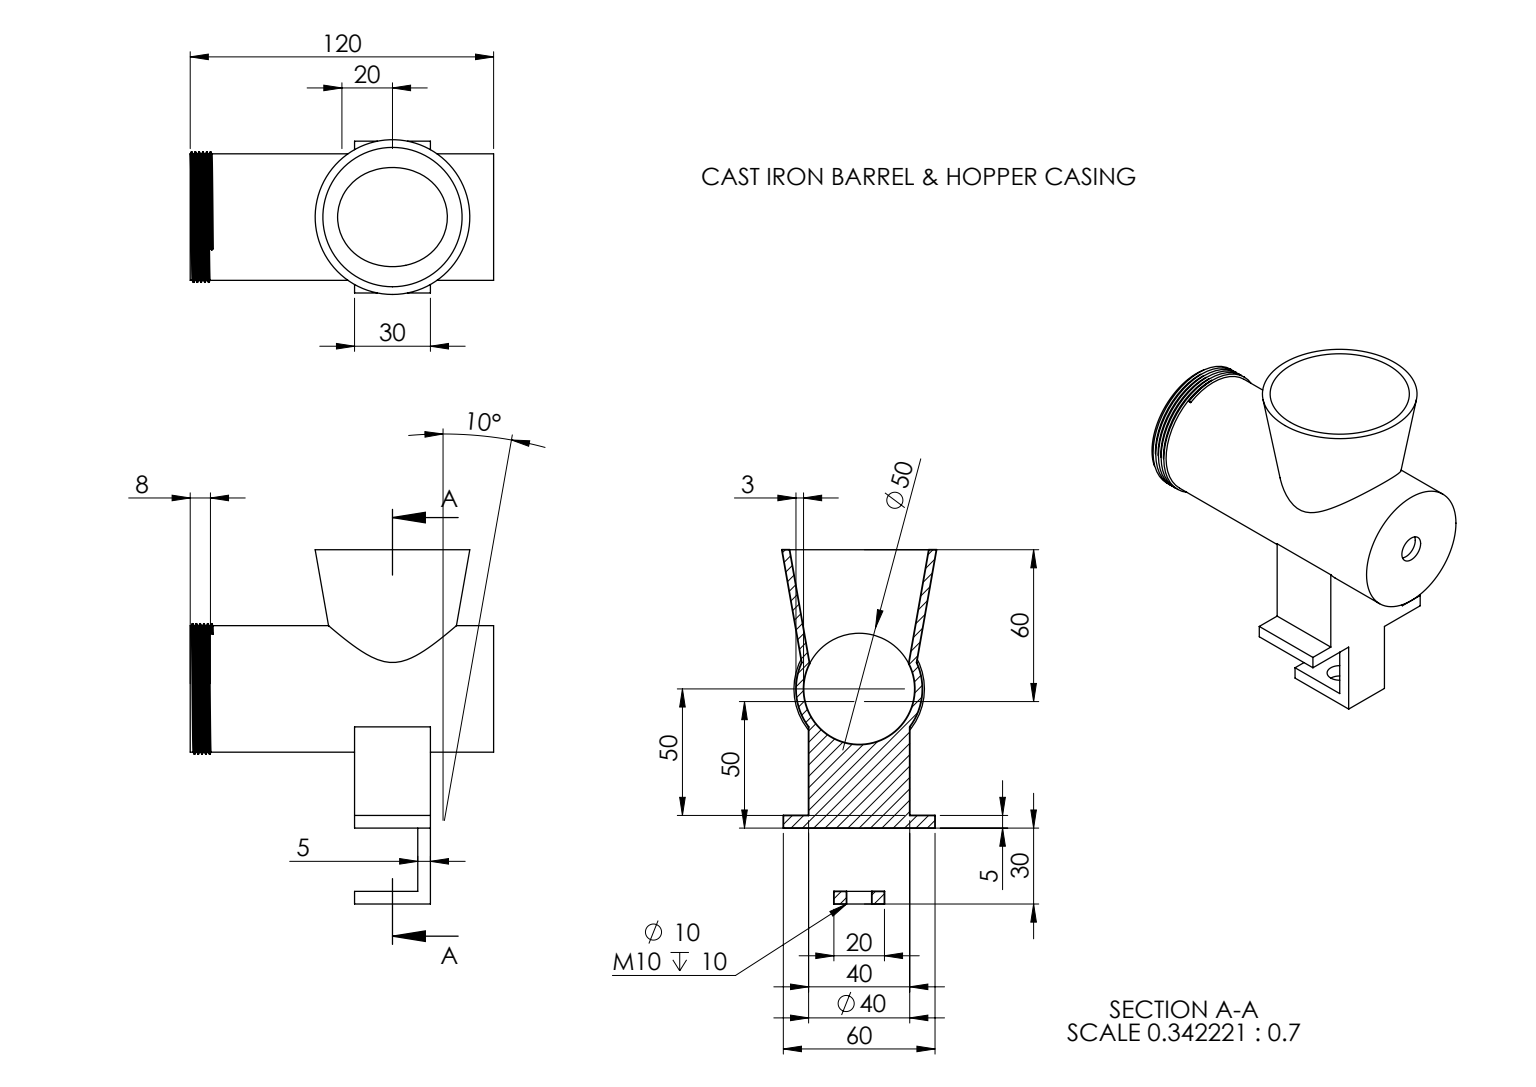
ISO-10303-21;
HEADER;
FILE_DESCRIPTION (('STEP AP214'),
    '1' );
FILE_NAME ('Cast Iron Barrel & Hopper Casing.step',
    '2026-10-22T10:02:39',
    ( '' ),
    ( '' ),
    'SwSTEP 2.0',
    'SolidWorks 2026',
    '' );
FILE_SCHEMA (( 'AUTOMOTIVE_DESIGN' ));
ENDSEC;

DATA;
#1=CARTESIAN_POINT ( 'NONE',  ( -15.00000000000000000, 55.00000000000000000, -20.00000000000000000 ) ) ;
#5=CARTESIAN_POINT ( 'NONE',  ( -21.63041020058595976, 76.92929161012460781, 1.799941901431467484 ) ) ;
#6=VECTOR ( 'NONE', #483, 1000.000000000000000 ) ;
#10=CARTESIAN_POINT ( 'NONE',  ( -15.00000000000000000, 5.000000000000000000, 20.00000000000000000 ) ) ;
#11=VERTEX_POINT ( 'NONE', #2092 ) ;
#13=CARTESIAN_POINT ( 'NONE',  ( -73.34375000204839523, 73.25176868561975141, -18.25176868561974430 ) ) ;
#30=VERTEX_POINT ( 'NONE', #8511 ) ;
#31=CARTESIAN_POINT ( 'NONE',  ( -76.62500000409677625, 55.00000000000000000, 24.99999999999999645 ) ) ;
#39=LINE ( 'NONE', #6477, #6145 ) ;
#41=CARTESIAN_POINT ( 'NONE',  ( -74.00000000204839523, 29.18810118750000981, 10.69163855873950020 ) ) ;
#44=CARTESIAN_POINT ( 'NONE',  ( -76.71875000204839523, 29.18810118750000271, 4.741568889096522788E-15 ) ) ;
#49=DIRECTION ( 'NONE',  ( 1.000000000000000000, 0.000000000000000000, 0.000000000000000000 ) ) ;
#50=LINE ( 'NONE', #11190, #9309 ) ;
#51=CARTESIAN_POINT ( 'NONE',  ( -78.03125000000002842, 79.99999999999992895, 10.35533905932734378 ) ) ;
#53=CARTESIAN_POINT ( 'NONE',  ( -79.25000000000000000, 55.00000000000000000, 24.99999999999999645 ) ) ;
#62=CARTESIAN_POINT ( 'NONE',  ( -19.12261397941723473, 74.85860496676178855, 9.489298872914485372 ) ) ;
#64=EDGE_CURVE ( 'NONE', #4200, #8679, #1605, .T. ) ;
#71=CARTESIAN_POINT ( 'NONE',  ( -71.59560441781462714, 80.81189881250000440, 6.916273779317701376 ) ) ;
#73=ADVANCED_FACE ( 'NONE', ( #817 ), #4433, .F. ) ;
#93=CARTESIAN_POINT ( 'NONE',  ( 9.999999999999994671, -24.99999999999999645, 10.00000000000000000 ) ) ;
#98=CARTESIAN_POINT ( 'NONE',  ( -71.75000000204838102, 80.81189881250000440, -10.69163855873948954 ) ) ;
#99=CARTESIAN_POINT ( 'NONE',  ( 3.371861548457865722E-15, 110.0000000000000000, -27.53333900685068869 ) ) ;
#101=CARTESIAN_POINT ( 'NONE',  ( 0.000000000000000000, -24.99999999999999645, -5.000000000000000000 ) ) ;
#104=ORIENTED_EDGE ( 'NONE', *, *, #11406, .F. ) ;
#105=CARTESIAN_POINT ( 'NONE',  ( -77.65625000204839523, 73.25176868561975141, -18.25176868561974430 ) ) ;
#107=CARTESIAN_POINT ( 'NONE',  ( 24.10175047695886619, 78.98596163070220655, -7.059706225875322261 ) ) ;
#109=VECTOR ( 'NONE', #311, 1000.000000000000000 ) ;
#111=EDGE_CURVE ( 'NONE', #9073, #8979, #3345, .T. ) ;
#112=DIRECTION ( 'NONE',  ( 0.000000000000000000, -0.000000000000000000, 1.000000000000000000 ) ) ;
#115=VECTOR ( 'NONE', #7085, 1000.000000000000000 ) ;
#116=CARTESIAN_POINT ( 'NONE',  ( -78.31250000000000000, 72.67766952966368876, -17.67766952966368876 ) ) ;
#120=DIRECTION ( 'NONE',  ( 1.000000000000000000, 0.000000000000000000, -0.000000000000000000 ) ) ;
#122=SHAPE_DEFINITION_REPRESENTATION ( #1837, #423 ) ;
#124=CARTESIAN_POINT ( 'NONE',  ( -10.64432325360710152, 68.67941443230903076, -17.23560473394323367 ) ) ;
#133=PRODUCT_DEFINITION ( 'UNKNOWN', '', #852, #2465 ) ;
#134=CARTESIAN_POINT ( 'NONE',  ( -76.71875000204839523, 29.18810118750000271, 4.741568889096522788E-15 ) ) ;
#135=CARTESIAN_POINT ( 'NONE',  ( -15.00000000000000355, 5.000000000000000000, -29.99999999999999289 ) ) ;
#138=ORIENTED_EDGE ( 'NONE', *, *, #9495, .F. ) ;
#140=EDGE_CURVE ( 'NONE', #7402, #8679, #2318, .T. ) ;
#147=CARTESIAN_POINT ( 'NONE',  ( -73.34375000409679046, 30.00000000000001421, 10.35533905932739174 ) ) ;
#148=DIRECTION ( 'NONE',  ( -1.000000000000000000, -0.000000000000000000, -0.000000000000000000 ) ) ;
#153=DIRECTION ( 'NONE',  ( 0.000000000000000000, -0.000000000000000000, 1.000000000000000000 ) ) ;
#160=ORIENTED_EDGE ( 'NONE', *, *, #1242, .F. ) ;
#164=FACE_BOUND ( 'NONE', #3650, .T. ) ;
#165=CARTESIAN_POINT ( 'NONE',  ( -12.37866201454132487, 69.98577131611273217, -20.01755997183146718 ) ) ;
#168=CARTESIAN_POINT ( 'NONE',  ( -78.59375000204839523, 55.00000000000000000, 25.81189881249999729 ) ) ;
#171=CARTESIAN_POINT ( 'NONE',  ( 3.392634454741613848, 65.79950035100726780, -22.54765914078175015 ) ) ;
#178=CARTESIAN_POINT ( 'NONE',  ( -15.00000000000000355, 0.000000000000000000, -29.99999999999999289 ) ) ;
#179=VECTOR ( 'NONE', #1295, 1000.000000000000000 ) ;
#182=FACE_OUTER_BOUND ( 'NONE', #3755, .T. ) ;
#187=CARTESIAN_POINT ( 'NONE',  ( -7.638500494831339971, 67.00046308197731548, 18.44294210305378456 ) ) ;
#191=FACE_OUTER_BOUND ( 'NONE', #2836, .T. ) ;
#193=VERTEX_POINT ( 'NONE', #2983 ) ;
#196=CARTESIAN_POINT ( 'NONE',  ( -78.68750000204839523, 65.69163855873949842, 25.81189881250000440 ) ) ;
#204=ORIENTED_EDGE ( 'NONE', *, *, #9495, .T. ) ;
#205=CARTESIAN_POINT ( 'NONE',  ( -71.93750000204838102, 44.30836144126049447, -25.81189881249999019 ) ) ;
#208=FACE_OUTER_BOUND ( 'NONE', #5773, .T. ) ;
#214=CARTESIAN_POINT ( 'NONE',  ( -75.87500000409677625, 55.00000000000000000, -24.99999999999999645 ) ) ;
#218=ORIENTED_EDGE ( 'NONE', *, *, #5065, .F. ) ;
#230=CARTESIAN_POINT ( 'NONE',  ( -71.84375000204838102, 73.25176868561975141, -18.25176868561974430 ) ) ;
#233=CARTESIAN_POINT ( 'NONE',  ( -76.06250000409679046, 37.32233047033631124, -17.67766952966368166 ) ) ;
#234=ORIENTED_EDGE ( 'NONE', *, *, #5652, .T. ) ;
#235=CARTESIAN_POINT ( 'NONE',  ( 23.67201755683229081, 78.62200754200915753, -8.225812365109568702 ) ) ;
#249=EDGE_LOOP ( 'NONE', ( #1338, #6982, #2879, #8696 ) ) ;
#254=CARTESIAN_POINT ( 'NONE',  ( -75.87500000204839523, 80.81189881250001861, 10.69163855873948599 ) ) ;
#259=ORIENTED_EDGE ( 'NONE', *, *, #6814, .T. ) ;
#261=CARTESIAN_POINT ( 'NONE',  ( -73.71875000204839523, 29.18810118750000271, 4.741568889096522788E-15 ) ) ;
#270=CARTESIAN_POINT ( 'NONE',  ( -76.34375000409679046, 30.00000000000001421, 10.35533905932739174 ) ) ;
#272=CARTESIAN_POINT ( 'NONE',  ( -72.06435441788595142, 79.99999999999991473, 6.698726029249561620 ) ) ;
#278=PLANE ( 'NONE',  #4388 ) ;
#279=CARTESIAN_POINT ( 'NONE',  ( -15.00000000000000000, -24.99999999999999645, 10.00000000000000000 ) ) ;
#292=CARTESIAN_POINT ( 'NONE',  ( -73.62500000204842365, 29.18810118750000626, -10.69163855873949309 ) ) ;
#294=DIRECTION ( 'NONE',  ( -1.000000000000000000, 0.000000000000000000, -0.000000000000000000 ) ) ;
#296=CARTESIAN_POINT ( 'NONE',  ( 0.000000000000000000, 0.000000000000000000, 10.00000000000000000 ) ) ;
#303=CARTESIAN_POINT ( 'NONE',  ( -77.28124999999998579, 30.00000000000000355, -10.35533905932738108 ) ) ;
#305=CARTESIAN_POINT ( 'NONE',  ( -77.00000000000000000, 55.00000000000000000, -24.99999999999999645 ) ) ;
#309=CARTESIAN_POINT ( 'NONE',  ( -2.905210441188253778, 65.30173033721455056, 19.43922460838591348 ) ) ;
#311=DIRECTION ( 'NONE',  ( 1.000000000000000000, 0.000000000000000000, 0.000000000000000000 ) ) ;
#312=ORIENTED_EDGE ( 'NONE', *, *, #8953, .F. ) ;
#313=DIRECTION ( 'NONE',  ( 0.000000000000000000, 0.000000000000000000, -1.000000000000000000 ) ) ;
#317=CARTESIAN_POINT ( 'NONE',  ( -73.90625000204839523, 36.74823131438026280, 18.25176868561974786 ) ) ;
#333=CARTESIAN_POINT ( 'NONE',  ( -72.31250000000007105, 72.67766952966360350, -17.67766952966359995 ) ) ;
#343=DIRECTION ( 'NONE',  ( 0.000000000000000000, 1.000000000000000000, 0.000000000000000000 ) ) ;
#346=CARTESIAN_POINT ( 'NONE',  ( -3.398726575883826762, 65.81855960629934543, 22.53824819929336698 ) ) ;
#350=CARTESIAN_POINT ( 'NONE',  ( -78.21875000409679046, 65.35533905932737753, 24.99999999999999645 ) ) ;
#352=CARTESIAN_POINT ( 'NONE',  ( 12.39308895597016047, 69.98013642987091032, -20.04675360703169318 ) ) ;
#355=AXIS2_PLACEMENT_3D ( 'NONE', #11527, #8791, #3333 ) ;
#360=CARTESIAN_POINT ( 'NONE',  ( -74.56250000000000000, 37.32233047033631124, 17.67766952966369232 ) ) ;
#367=DIRECTION ( 'NONE',  ( -0.000000000000000000, -1.000000000000000000, -0.000000000000000000 ) ) ;
#372=CARTESIAN_POINT ( 'NONE',  ( 39.99999999999999289, 55.00000000000000000, 0.000000000000000000 ) ) ;
#373=CARTESIAN_POINT ( 'NONE',  ( -75.96875000204839523, 73.25176868561975141, 18.25176868561974075 ) ) ;
#377=CARTESIAN_POINT ( 'NONE',  ( -75.03125000204839523, 36.74823131438024859, -18.25176868561973720 ) ) ;
#381=CARTESIAN_POINT ( 'NONE',  ( -15.00000000000000355, 0.000000000000000000, 30.00000000000000711 ) ) ;
#384=CARTESIAN_POINT ( 'NONE',  ( -74.00000000204839523, 44.30836144126052289, 25.81189881250000795 ) ) ;
#385=CARTESIAN_POINT ( 'NONE',  ( -80.00000000000000000, 55.00000000000000000, 24.99999999999999645 ) ) ;
#388=VERTEX_POINT ( 'NONE', #6780 ) ;
#399=CIRCLE ( 'NONE', #11681, 24.99999999999999645 ) ;
#408=CARTESIAN_POINT ( 'NONE',  ( -75.31250000204839523, 29.18810118750000981, 10.69163855873950020 ) ) ;
#412=CARTESIAN_POINT ( 'NONE',  ( -77.65625000409677625, 30.00000000000000355, -10.35533905932738108 ) ) ;
#419=CARTESIAN_POINT ( 'NONE',  ( -73.71875000000005684, 79.99999999999987210, -10.35533905932732424 ) ) ;
#421=CARTESIAN_POINT ( 'NONE',  ( -77.09374999999998579, 44.64466094067260826, -24.99999999999998934 ) ) ;
#423=SHAPE_REPRESENTATION ( 'Cast Iron Barrel & Hopper Casing', ( #4738 ), #3015 ) ;
#426=EDGE_CURVE ( 'NONE', #7502, #11, #9516, .T. ) ;
#427=ADVANCED_FACE ( 'NONE', ( #5819, #10408 ), #5935, .F. ) ;
#431=CARTESIAN_POINT ( 'NONE',  ( 10.64984185237921466, 68.68279778901450072, -17.23294504368761793 ) ) ;
#433=CARTESIAN_POINT ( 'NONE',  ( -78.87500000204839523, 65.69163855873949842, 25.81189881250000084 ) ) ;
#436=CARTESIAN_POINT ( 'NONE',  ( -72.68750000204839523, 65.69163855873949842, 25.81189881250000440 ) ) ;
#437=ADVANCED_FACE ( 'NONE', ( #8976 ), #2509, .T. ) ;
#454=CARTESIAN_POINT ( 'NONE',  ( -73.62500000409677625, 55.00000000000000000, 24.99999999999999645 ) ) ;
#464=FACE_OUTER_BOUND ( 'NONE', #2972, .T. ) ;
#465=DIRECTION ( 'NONE',  ( 0.000000000000000000, 0.000000000000000000, 1.000000000000000000 ) ) ;
#466=CARTESIAN_POINT ( 'NONE',  ( -77.09375000204839523, 55.00000000000000000, 25.81189881249999729 ) ) ;
#467=CARTESIAN_POINT ( 'NONE',  ( -11.05058114698192107, 69.12285606448547526, 20.64999657351882689 ) ) ;
#470=CARTESIAN_POINT ( 'NONE',  ( -76.34375000409680467, 30.00000000000001421, 10.35533905932739174 ) ) ;
#474=CARTESIAN_POINT ( 'NONE',  ( -75.21875000000007105, 79.99999999999990052, -10.35533905932733134 ) ) ;
#481=CARTESIAN_POINT ( 'NONE',  ( -72.21875000000001421, 80.00000000000001421, -10.35533905932737753 ) ) ;
#483=DIRECTION ( 'NONE',  ( -0.000000000000000000, -0.000000000000000000, -1.000000000000000000 ) ) ;
#485=EDGE_CURVE ( 'NONE', #7813, #9573, #2446, .T. ) ;
#488=LINE ( 'NONE', #11560, #10630 ) ;
#492=CARTESIAN_POINT ( 'NONE',  ( 21.70367235178696319, 76.99085433373973331, 0.7325029477543631984 ) ) ;
#493=CARTESIAN_POINT ( 'NONE',  ( -77.84375000204839523, 73.25176868561975141, -18.25176868561974430 ) ) ;
#494=VERTEX_POINT ( 'NONE', #7845 ) ;
#495=CARTESIAN_POINT ( 'NONE',  ( -72.03125000204839523, 36.74823131438024859, -18.25176868561973720 ) ) ;
#500=ORIENTED_EDGE ( 'NONE', *, *, #3520, .F. ) ;
#502=ORIENTED_EDGE ( 'NONE', *, *, #10815, .T. ) ;
#523=CARTESIAN_POINT ( 'NONE',  ( -79.06250000204840944, 80.81189881250000440, -10.69163855873948954 ) ) ;
#524=CARTESIAN_POINT ( 'NONE',  ( -1.708601562010274133, 65.50638515368892456, 22.68572929305231867 ) ) ;
#526=ORIENTED_EDGE ( 'NONE', *, *, #1693, .F. ) ;
#527=CARTESIAN_POINT ( 'NONE',  ( -74.37500000409677625, 55.00000000000000000, -24.99999999999999645 ) ) ;
#530=AXIS2_PLACEMENT_3D ( 'NONE', #8639, #9703, #5223 ) ;
#538=CARTESIAN_POINT ( 'NONE',  ( -74.75000000000000000, 55.00000000000000000, 24.99999999999999645 ) ) ;
#542=EDGE_CURVE ( 'NONE', #5255, #5411, #11153, .T. ) ;
#546=VERTEX_POINT ( 'NONE', #9861 ) ;
#547=CARTESIAN_POINT ( 'NONE',  ( 2.917962331683024768, 65.29045701389995315, -19.44540138122387773 ) ) ;
#549=ORIENTED_EDGE ( 'NONE', *, *, #6671, .F. ) ;
#552=CARTESIAN_POINT ( 'NONE',  ( -75.40625000409677625, 80.00000000000001421, 10.35533905932737397 ) ) ;
#565=CARTESIAN_POINT ( 'NONE',  ( -74.18750000204838102, 44.30836144126053000, 25.81189881250000795 ) ) ;
#580=CARTESIAN_POINT ( 'NONE',  ( -77.46875000204839523, 80.81189881250000440, -1.580522963032174394E-15 ) ) ;
#584=CARTESIAN_POINT ( 'NONE',  ( -75.12500000409677625, 55.00000000000000000, 24.99999999999999645 ) ) ;
#585=DIRECTION ( 'NONE',  ( -1.000000000000000000, -0.000000000000000000, -0.000000000000000000 ) ) ;
#586=CARTESIAN_POINT ( 'NONE',  ( -71.56250000409677625, 37.32233047033631124, -17.67766952966368166 ) ) ;
#592=AXIS2_PLACEMENT_3D ( 'NONE', #1916, #1680, #10056 ) ;
#594=CARTESIAN_POINT ( 'NONE',  ( 39.99999999999999289, 55.00000000000000000, 0.000000000000000000 ) ) ;
#598=CARTESIAN_POINT ( 'NONE',  ( -78.03125000204838102, 55.00000000000000000, -25.81189881249999729 ) ) ;
#610=VECTOR ( 'NONE', #11628, 1000.000000000000000 ) ;
#611=CARTESIAN_POINT ( 'NONE',  ( 12.31292331232940640, 69.75642766769821890, 16.32415115763334867 ) ) ;
#612=CARTESIAN_POINT ( 'NONE',  ( -72.12500000204839523, 44.30836144126049447, -25.81189881249999019 ) ) ;
#625=CARTESIAN_POINT ( 'NONE',  ( -77.75000000204839523, 80.81189881250001861, -10.69163855873949132 ) ) ;
#630=( BOUNDED_CURVE ( )  B_SPLINE_CURVE ( 2, ( #7577, #9479, #6681, #10311, #8593, #2108, #3973, #5782, #1209 ),
 .UNSPECIFIED., .F., .T. ) 
 B_SPLINE_CURVE_WITH_KNOTS ( ( 3, 2, 2, 2, 3 ),
 ( 0.7129436809910058015, 0.7327527857159548130, 0.7525618904409037135, 0.7723709951658527251, 0.7921800998908017366 ),
 .UNSPECIFIED. ) 
 CURVE ( )  GEOMETRIC_REPRESENTATION_ITEM ( )  RATIONAL_B_SPLINE_CURVE ( ( 1.000000000000000000, 0.9238795325112866275, 1.000000000000000000, 0.9238795325112866275, 1.000000000000000000, 0.9238795325112866275, 1.000000000000000000, 0.9238795325112866275, 1.000000000000000000 ) ) 
 REPRESENTATION_ITEM ( '' )  );
#633=CARTESIAN_POINT ( 'NONE',  ( 0.000000000000000000, -30.00000000000000000, 0.000000000000000000 ) ) ;
#644=CARTESIAN_POINT ( 'NONE',  ( -71.37500000409677625, 55.00000000000000000, -24.99999999999999645 ) ) ;
#648=ORIENTED_EDGE ( 'NONE', *, *, #111, .F. ) ;
#654=CARTESIAN_POINT ( 'NONE',  ( -74.84375000204839523, 73.25176868561975141, -18.25176868561974430 ) ) ;
#655=CYLINDRICAL_SURFACE ( 'NONE', #8229, 5.000000000000000000 ) ;
#661=CARTESIAN_POINT ( 'NONE',  ( -71.34302368722835297, 77.35376350879521112, 12.90594348738575903 ) ) ;
#664=CARTESIAN_POINT ( 'NONE',  ( 20.82597707344048743, 76.25689989831184334, -5.711711607058635565 ) ) ;
#665=CARTESIAN_POINT ( 'NONE',  ( -71.93750000204838102, 65.69163855873948421, -25.81189881250000084 ) ) ;
#668=EDGE_CURVE ( 'NONE', #7145, #5117, #992, .T. ) ;
#681=CARTESIAN_POINT ( 'NONE',  ( -79.25000000204838102, 80.81189881250001861, -10.69163855873949132 ) ) ;
#696=FACE_OUTER_BOUND ( 'NONE', #7625, .T. ) ;
#698=ORIENTED_EDGE ( 'NONE', *, *, #6458, .F. ) ;
#699=CARTESIAN_POINT ( 'NONE',  ( -74.28125000409676204, 65.35533905932737753, -24.99999999999999645 ) ) ;
#706=CIRCLE ( 'NONE', #5497, 5.000000000000000000 ) ;
#707=CARTESIAN_POINT ( 'NONE',  ( -15.00000000000000355, 5.000000000000000000, 30.00000000000000711 ) ) ;
#708=CARTESIAN_POINT ( 'NONE',  ( -71.53052369147287948, 77.35376373433385311, 12.90594309674112772 ) ) ;
#711=CARTESIAN_POINT ( 'NONE',  ( -76.15625000204838102, 80.81189881250000440, -1.580522963032174394E-15 ) ) ;
#716=CARTESIAN_POINT ( 'NONE',  ( 23.71418293028490609, 78.65541738657648807, 8.238313537303401546 ) ) ;
#718=DIRECTION ( 'NONE',  ( 0.000000000000000000, 1.000000000000000000, 0.000000000000000000 ) ) ;
#720=AXIS2_PLACEMENT_3D ( 'NONE', #11548, #3350, #6967 ) ;
#722=CARTESIAN_POINT ( 'NONE',  ( -74.65625000204838102, 80.81189881250000440, -1.580522963032174394E-15 ) ) ;
#726=EDGE_CURVE ( 'NONE', #10529, #7325, #4652, .T. ) ;
#736=ORIENTED_EDGE ( 'NONE', *, *, #5482, .T. ) ;
#738=CARTESIAN_POINT ( 'NONE',  ( -77.46875000204839523, 73.25176868561975141, 18.25176868561974075 ) ) ;
#744=ORIENTED_EDGE ( 'NONE', *, *, #1054, .T. ) ;
#752=CARTESIAN_POINT ( 'NONE',  ( 0.000000000000000000, 0.000000000000000000, 0.000000000000000000 ) ) ;
#755=EDGE_LOOP ( 'NONE', ( #5969, #1527, #204, #6990 ) ) ;
#756=CARTESIAN_POINT ( 'NONE',  ( -76.43750000000005684, 72.67766952966361771, 17.67766952966361771 ) ) ;
#757=DIRECTION ( 'NONE',  ( 0.000000000000000000, 0.000000000000000000, -1.000000000000000000 ) ) ;
#766=VECTOR ( 'NONE', #5661, 1000.000000000000000 ) ;
#768=CARTESIAN_POINT ( 'NONE',  ( -76.53125000204838102, 55.00000000000000000, -25.81189881249999729 ) ) ;
#772=AXIS2_PLACEMENT_3D ( 'NONE', #6466, #10095, #5562 ) ;
#778=CARTESIAN_POINT ( 'NONE',  ( 1.837682338809236926, 65.11633786365413812, -19.53622259640674130 ) ) ;
#787=CARTESIAN_POINT ( 'NONE',  ( 39.99999999999999289, 55.00000000000000000, -24.99999999999999645 ) ) ;
#791=ORIENTED_EDGE ( 'NONE', *, *, #3827, .T. ) ;
#796=FACE_OUTER_BOUND ( 'NONE', #4135, .T. ) ;
#800=ORIENTED_EDGE ( 'NONE', *, *, #878, .F. ) ;
#812=CARTESIAN_POINT ( 'NONE',  ( -75.50000000000001421, 54.99999999999944578, -24.99999999999999645 ) ) ;
#815=CARTESIAN_POINT ( 'NONE',  ( -77.00000000000000000, 55.00000000000000000, -24.99999999999999645 ) ) ;
#816=DIRECTION ( 'NONE',  ( -1.000000000000000000, 0.000000000000000000, -0.000000000000000000 ) ) ;
#817=FACE_OUTER_BOUND ( 'NONE', #7666, .T. ) ;
#824=CARTESIAN_POINT ( 'NONE',  ( -71.95822497812569907, 74.53807824654330716, 16.15905817987090032 ) ) ;
#827=CARTESIAN_POINT ( 'NONE',  ( -76.81250000204839523, 29.18810118750000981, 10.69163855873950020 ) ) ;
#829=CARTESIAN_POINT ( 'NONE',  ( 5.447911505823581635, 66.41754438690165330, 22.24099615069902569 ) ) ;
#831=AXIS2_PLACEMENT_3D ( 'NONE', #7959, #7072, #7186 ) ;
#841=DIRECTION ( 'NONE',  ( -1.000000000000000000, -0.000000000000000000, -0.000000000000000000 ) ) ;
#845=CARTESIAN_POINT ( 'NONE',  ( -21.70513237093992132, 76.99208176644971502, 0.6955368305833549147 ) ) ;
#847=VERTEX_POINT ( 'NONE', #8429 ) ;
#851=CARTESIAN_POINT ( 'NONE',  ( -72.12500000204839523, 44.30836144126050158, -25.81189881249999374 ) ) ;
#852=PRODUCT_DEFINITION_FORMATION_WITH_SPECIFIED_SOURCE ( 'ANY', '', #3760, .NOT_KNOWN. ) ;
#859=DIRECTION ( 'NONE',  ( -0.000000000000000000, 1.000000000000000000, 0.000000000000000000 ) ) ;
#878=EDGE_CURVE ( 'NONE', #7673, #884, #5469, .T. ) ;
#883=CARTESIAN_POINT ( 'NONE',  ( -72.96875000204838102, 73.25176868561975141, 18.25176868561974075 ) ) ;
#884=VERTEX_POINT ( 'NONE', #10274 ) ;
#885=VECTOR ( 'NONE', #3491, 1000.000000000000000 ) ;
#886=CARTESIAN_POINT ( 'NONE',  ( -75.03125000204839523, 36.74823131438024859, -18.25176868561973720 ) ) ;
#887=ORIENTED_EDGE ( 'NONE', *, *, #6671, .T. ) ;
#888=CARTESIAN_POINT ( 'NONE',  ( 18.41792582001188805, 74.34136002823915135, 15.84364092613776975 ) ) ;
#889=VECTOR ( 'NONE', #6874, 1000.000000000000000 ) ;
#892=CARTESIAN_POINT ( 'NONE',  ( -79.15625000000001421, 44.64466094067263668, 24.99999999999997513 ) ) ;
#894=VECTOR ( 'NONE', #2900, 1000.000000000000000 ) ;
#896=VERTEX_POINT ( 'NONE', #10448 ) ;
#904=CARTESIAN_POINT ( 'NONE',  ( -18.37414261478594213, 74.25662752951258483, -10.65766454279107478 ) ) ;
#907=PLANE ( 'NONE',  #10710 ) ;
#910=CARTESIAN_POINT ( 'NONE',  ( -71.84375000204838102, 73.25176868561975141, -18.25176868561974430 ) ) ;
#919=B_SPLINE_CURVE_WITH_KNOTS ( 'NONE', 3,
 ( #8394, #9528, #1074, #10301 ),
 .UNSPECIFIED., .F., .F.,
 ( 4, 4 ),
 ( 0.000000000000000000, 1.000000000000000000 ),
 .UNSPECIFIED. ) ;
#928=VECTOR ( 'NONE', #3584, 1000.000000000000000 ) ;
#937=CARTESIAN_POINT ( 'NONE',  ( -74.93750000000007105, 72.67766952966361771, 17.67766952966360350 ) ) ;
#939=CARTESIAN_POINT ( 'NONE',  ( -77.37500000409677625, 55.00000000000000000, -24.99999999999999645 ) ) ;
#940=EDGE_LOOP ( 'NONE', ( #4887, #4146, #3980, #10315 ) ) ;
#942=CARTESIAN_POINT ( 'NONE',  ( 2.400054171417768487E-15, 64.99605696851786263, -19.59792961213366169 ) ) ;
#944=CARTESIAN_POINT ( 'NONE',  ( -73.34375000204839523, 73.25176868561975141, -18.25176868561974430 ) ) ;
#948=ADVANCED_FACE ( 'NONE', ( #3549 ), #2653, .T. ) ;
#949=CARTESIAN_POINT ( 'NONE',  ( -78.68750000204839523, 65.69163855873949842, 25.81189881250000440 ) ) ;
#954=FACE_OUTER_BOUND ( 'NONE', #6624, .T. ) ;
#962=CARTESIAN_POINT ( 'NONE',  ( -79.43750000000001421, 72.67766952966368876, 17.67766952966368521 ) ) ;
#969=AXIS2_PLACEMENT_3D ( 'NONE', #3189, #10486, #2290 ) ;
#976=CARTESIAN_POINT ( 'NONE',  ( -78.21875000204839523, 29.18810118750000271, 4.741568889096522788E-15 ) ) ;
#988=EDGE_LOOP ( 'NONE', ( #8464, #10923 ) ) ;
#992=LINE ( 'NONE', #1888, #5063 ) ;
#996=EDGE_CURVE ( 'NONE', #9989, #2344, #8449, .T. ) ;
#1005=CARTESIAN_POINT ( 'NONE',  ( -73.06250000204842365, 80.81189881250000440, 10.69163855873948243 ) ) ;
#1008=CARTESIAN_POINT ( 'NONE',  ( -71.48947498017410851, 75.17259594761931396, 16.68383898576512081 ) ) ;
#1011=CARTESIAN_POINT ( 'NONE',  ( -79.15625000204839523, 73.25176868561975141, -18.25176868561974430 ) ) ;
#1012=ORIENTED_EDGE ( 'NONE', *, *, #2580, .F. ) ;
#1015=( BOUNDED_CURVE ( )  B_SPLINE_CURVE ( 2, ( #2066, #9372, #1946, #10329, #7411, #9254, #6516, #3925, #11036 ),
 .UNSPECIFIED., .F., .T. ) 
 B_SPLINE_CURVE_WITH_KNOTS ( ( 3, 2, 2, 2, 3 ),
 ( 0.6666666666666671848, 0.6875000000000005551, 0.7083333333333339255, 0.7291666666666672958, 0.7500000000000006661 ),
 .UNSPECIFIED. ) 
 CURVE ( )  GEOMETRIC_REPRESENTATION_ITEM ( )  RATIONAL_B_SPLINE_CURVE ( ( 0.9999999999999980016, 0.9238795325112887369, 1.000000000000000000, 0.9238795325112867385, 1.000000000000000000, 0.9238795325112867385, 1.000000000000000000, 0.9238795325112842960, 1.000000000000002442 ) ) 
 REPRESENTATION_ITEM ( '' )  );
#1019=CARTESIAN_POINT ( 'NONE',  ( -78.96875000000000000, 30.00000000000001421, 10.35533905932739174 ) ) ;
#1021=CARTESIAN_POINT ( 'NONE',  ( 39.99999999999999289, 55.00000000000000000, 0.000000000000000000 ) ) ;
#1024=EDGE_CURVE ( 'NONE', #10896, #8154, #9201, .T. ) ;
#1026=CARTESIAN_POINT ( 'NONE',  ( -19.59385640182016530, 75.24237086212529846, -8.623108768566876137 ) ) ;
#1027=CARTESIAN_POINT ( 'NONE',  ( -71.37500000409677625, 55.00000000000000000, -24.99999999999999645 ) ) ;
#1029=CARTESIAN_POINT ( 'NONE',  ( 0.000000000000000000, 0.000000000000000000, -10.00000000000000000 ) ) ;
#1035=CARTESIAN_POINT ( 'NONE',  ( -77.37500000204838102, 80.81189881250001861, 10.69163855873948599 ) ) ;
#1041=CARTESIAN_POINT ( 'NONE',  ( -72.78125000204839523, 73.25176868561975141, 18.25176868561974075 ) ) ;
#1051=FACE_OUTER_BOUND ( 'NONE', #755, .T. ) ;
#1052=CYLINDRICAL_SURFACE ( 'NONE', #5002, 24.99999999999999645 ) ;
#1054=EDGE_CURVE ( 'NONE', #2054, #1879, #1860, .T. ) ;
#1055=FACE_OUTER_BOUND ( 'NONE', #4597, .T. ) ;
#1062=UNCERTAINTY_MEASURE_WITH_UNIT (LENGTH_MEASURE( 1.000000000000000082E-05 ), #8594, 'distance_accuracy_value', 'NONE');
#1066=CARTESIAN_POINT ( 'NONE',  ( -73.62500000204839523, 44.30836144126050158, -25.81189881249999374 ) ) ;
#1069=CARTESIAN_POINT ( 'NONE',  ( -77.46875000204839523, 80.81189881250000440, -1.580522963032174394E-15 ) ) ;
#1074=CARTESIAN_POINT ( 'NONE',  ( -71.46802368722833876, 77.35376350879521112, 12.90594348738575903 ) ) ;
#1087=CARTESIAN_POINT ( 'NONE',  ( -2.899087953157023723, 65.30046538299916392, -19.43989248047692442 ) ) ;
#1096=CARTESIAN_POINT ( 'NONE',  ( -79.34375000204839523, 55.00000000000000000, -25.81189881249999729 ) ) ;
#1121=ORIENTED_EDGE ( 'NONE', *, *, #9294, .F. ) ;
#1125=FACE_OUTER_BOUND ( 'NONE', #2753, .T. ) ;
#1126=CARTESIAN_POINT ( 'NONE',  ( -72.68750000204839523, 44.30836144126053000, 25.81189881250000795 ) ) ;
#1129=CARTESIAN_POINT ( 'NONE',  ( -78.03125000409677625, 44.64466094067262958, 25.00000000000001066 ) ) ;
#1130=AXIS2_PLACEMENT_3D ( 'NONE', #6175, #8085, #11658 ) ;
#1132=CARTESIAN_POINT ( 'NONE',  ( 25.03499957223221628, 79.78147775635788719, -3.407189920745893108 ) ) ;
#1139=CARTESIAN_POINT ( 'NONE',  ( -78.40625000000000000, 65.35533905932737753, -24.99999999999999645 ) ) ;
#1141=DIRECTION ( 'NONE',  ( 0.000000000000000000, 0.4999997706924120822, -0.8660255361751958425 ) ) ;
#1143=EDGE_CURVE ( 'NONE', #3987, #494, #8398, .T. ) ;
#1146=ADVANCED_FACE ( 'NONE', ( #182 ), #11647, .F. ) ;
#1151=DIRECTION ( 'NONE',  ( 1.000000000000000000, 0.000000000000000000, 0.000000000000000000 ) ) ;
#1153=VERTEX_POINT ( 'NONE', #101 ) ;
#1156=CARTESIAN_POINT ( 'NONE',  ( -74.37500000204838102, 80.81189881250001861, 10.69163855873948599 ) ) ;
#1168=EDGE_CURVE ( 'NONE', #8716, #7813, #8354, .T. ) ;
#1175=CARTESIAN_POINT ( 'NONE',  ( -15.00000000000000355, 0.000000000000000000, 30.00000000000000711 ) ) ;
#1177=ORIENTED_EDGE ( 'NONE', *, *, #5340, .T. ) ;
#1193=CARTESIAN_POINT ( 'NONE',  ( -22.63432272110139110, 77.75090647838392499, 10.39239001733118783 ) ) ;
#1196=CARTESIAN_POINT ( 'NONE',  ( -71.40810441781462714, 80.81189881250000440, 6.916273779317701376 ) ) ;
#1198=CARTESIAN_POINT ( 'NONE',  ( 24.58810204984513348, 79.39961546340161647, -5.461861930764240647 ) ) ;
#1206=LINE ( 'NONE', #5960, #6 ) ;
#1209=CARTESIAN_POINT ( 'NONE',  ( -72.50000000000000000, 55.00000000000000000, -24.99999999999999645 ) ) ;
#1213=CARTESIAN_POINT ( 'NONE',  ( -78.78125000204838102, 55.00000000000000000, 25.81189881249999729 ) ) ;
#1216=CARTESIAN_POINT ( 'NONE',  ( -71.56250000204838102, 80.81189881250001861, -10.69163855873949132 ) ) ;
#1219=CARTESIAN_POINT ( 'NONE',  ( -77.93750000409679046, 37.32233047033631124, 17.67766952966369232 ) ) ;
#1220=EDGE_LOOP ( 'NONE', ( #9174, #10799, #9543, #8141, #4587, #5459, #10657, #5694, #7579, #2967, #800, #10288, #2333, #138 ) ) ;
#1225=ADVANCED_FACE ( 'NONE', ( #11306, #3116 ), #6782, .T. ) ;
#1242=EDGE_CURVE ( 'NONE', #9881, #10478, #2712, .T. ) ;
#1245=CARTESIAN_POINT ( 'NONE',  ( -2.976011536945806224, 65.72704692019560468, 22.58178635561741032 ) ) ;
#1249=CARTESIAN_POINT ( 'NONE',  ( -77.93750000409679046, 37.32233047033631124, 17.67766952966369232 ) ) ;
#1259=CARTESIAN_POINT ( 'NONE',  ( -76.15624999999998579, 44.64466094067262958, 25.00000000000001066 ) ) ;
#1261=( BOUNDED_CURVE ( )  B_SPLINE_CURVE ( 2, ( #11742, #1796, #8158, #4329, #4505, #8218, #3605, #10900, #9834 ),
 .UNSPECIFIED., .F., .T. ) 
 B_SPLINE_CURVE_WITH_KNOTS ( ( 3, 2, 2, 2, 3 ),
 ( 0.1666666666666667962, 0.1875000000000001665, 0.2083333333333335369, 0.2291666666666668517, 0.2500000000000002220 ),
 .UNSPECIFIED. ) 
 CURVE ( )  GEOMETRIC_REPRESENTATION_ITEM ( )  RATIONAL_B_SPLINE_CURVE ( ( 0.9999999999999994449, 0.9238795325112872936, 1.000000000000000000, 0.9238795325112867385, 1.000000000000000000, 0.9238795325112867385, 1.000000000000000000, 0.9238795325112859613, 1.000000000000000888 ) ) 
 REPRESENTATION_ITEM ( '' )  );
#1267=CARTESIAN_POINT ( 'NONE',  ( 14.99999999999999645, 5.000000000000000000, 30.00000000000000711 ) ) ;
#1272=CARTESIAN_POINT ( 'NONE',  ( -76.43750000204838102, 65.69163855873948421, -25.81189881250000084 ) ) ;
#1276=CARTESIAN_POINT ( 'NONE',  ( -73.34375000204839523, 55.00000000000000000, -25.81189881249999729 ) ) ;
#1279=AXIS2_PLACEMENT_3D ( 'NONE', #7664, #3219, #3045 ) ;
#1283=ORIENTED_EDGE ( 'NONE', *, *, #7410, .T. ) ;
#1284=CARTESIAN_POINT ( 'NONE',  ( -72.31250000204839523, 29.18810118750000981, 10.69163855873950020 ) ) ;
#1287=ORIENTED_EDGE ( 'NONE', *, *, #3917, .F. ) ;
#1295=DIRECTION ( 'NONE',  ( -1.000000000000000000, -0.000000000000000000, -0.000000000000000000 ) ) ;
#1299=LINE ( 'NONE', #4722, #6694 ) ;
#1309=CARTESIAN_POINT ( 'NONE',  ( -75.40625000204839523, 36.74823131438026280, 18.25176868561974786 ) ) ;
#1310=CARTESIAN_POINT ( 'NONE',  ( -24.23439331329375790, 79.09827848464085776, -6.702477181294344000 ) ) ;
#1313=CARTESIAN_POINT ( 'NONE',  ( -77.84375000409677625, 30.00000000000001421, 10.35533905932739174 ) ) ;
#1314=ORIENTED_EDGE ( 'NONE', *, *, #7805, .F. ) ;
#1317=DIRECTION ( 'NONE',  ( -1.000000000000000000, 0.000000000000000000, -0.000000000000000000 ) ) ;
#1326=CARTESIAN_POINT ( 'NONE',  ( -72.50000000000000000, 55.00000000000000000, -24.99999999999999645 ) ) ;
#1337=ADVANCED_FACE ( 'NONE', ( #696 ), #9747, .T. ) ;
#1338=ORIENTED_EDGE ( 'NONE', *, *, #2939, .F. ) ;
#1339=CARTESIAN_POINT ( 'NONE',  ( 10.64825151755819022, 68.66818062749433693, 17.26560489676726462 ) ) ;
#1341=CARTESIAN_POINT ( 'NONE',  ( -75.68750000204838102, 44.30836144126052289, 25.81189881250000795 ) ) ;
#1344=CARTESIAN_POINT ( 'NONE',  ( -75.21875000204839523, 29.18810118750000271, 4.741568889096522788E-15 ) ) ;
#1356=LINE ( 'NONE', #5861, #6889 ) ;
#1368=DIRECTION ( 'NONE',  ( 0.000000000000000000, 0.000000000000000000, 1.000000000000000000 ) ) ;
#1374=CARTESIAN_POINT ( 'NONE',  ( -78.50000000204842365, 44.30836144126052289, 25.81189881250000795 ) ) ;
#1375=CARTESIAN_POINT ( 'NONE',  ( -8.896007692468192118, 67.93420365865686961, 21.39919931194891944 ) ) ;
#1377=ORIENTED_EDGE ( 'NONE', *, *, #7805, .T. ) ;
#1379=CARTESIAN_POINT ( 'NONE',  ( -76.53125000409677625, 44.64466094067262958, 25.00000000000001066 ) ) ;
#1383=DIRECTION ( 'NONE',  ( 1.000000000000000000, 0.000000000000000000, 0.000000000000000000 ) ) ;
#1387=CARTESIAN_POINT ( 'NONE',  ( -73.62500000000008527, 79.99999999999987210, -1.530808498934183435E-15 ) ) ;
#1390=CARTESIAN_POINT ( 'NONE',  ( -74.28125000000000000, 30.00000000000000355, -10.35533905932738108 ) ) ;
#1397=ORIENTED_EDGE ( 'NONE', *, *, #5431, .T. ) ;
#1398=CARTESIAN_POINT ( 'NONE',  ( 20.45981033141799088, 75.95367107335623302, 6.713009951748246884 ) ) ;
#1410=ADVANCED_FACE ( 'NONE', ( #5150 ), #2091, .T. ) ;
#1425=ORIENTED_EDGE ( 'NONE', *, *, #4742, .T. ) ;
#1429=CARTESIAN_POINT ( 'NONE',  ( -76.90625000204839523, 36.74823131438026280, 18.25176868561974786 ) ) ;
#1431=CARTESIAN_POINT ( 'NONE',  ( -4.637059203130386109, 66.15064323337712437, 22.37599513459590028 ) ) ;
#1433=ORIENTED_EDGE ( 'NONE', *, *, #3169, .T. ) ;
#1434=CARTESIAN_POINT ( 'NONE',  ( -75.03125000409677625, 44.64466094067262958, 25.00000000000001066 ) ) ;
#1438=CARTESIAN_POINT ( 'NONE',  ( -75.40625000000007105, 65.35533905932709331, -25.00000000000012790 ) ) ;
#1444=CARTESIAN_POINT ( 'NONE',  ( -74.09375000000000000, 44.64466094067260826, -24.99999999999998934 ) ) ;
#1447=DIRECTION ( 'NONE',  ( 0.000000000000000000, 0.000000000000000000, -1.000000000000000000 ) ) ;
#1456=CARTESIAN_POINT ( 'NONE',  ( 11.22402665386259280, 69.04425390357937431, -16.94073621750904124 ) ) ;
#1457=CARTESIAN_POINT ( 'NONE',  ( -75.40625000204838102, 29.18810118750000271, 4.741568889096522788E-15 ) ) ;
#1458=ORIENTED_EDGE ( 'NONE', *, *, #7447, .T. ) ;
#1463=CARTESIAN_POINT ( 'NONE',  ( -75.87500000409677625, 55.00000000000000000, -24.99999999999999645 ) ) ;
#1480=CYLINDRICAL_SURFACE ( 'NONE', #355, 24.99999999999999645 ) ;
#1481=AXIS2_PLACEMENT_3D ( 'NONE', #1029, #4878, #11267 ) ;
#1487=DIRECTION ( 'NONE',  ( 1.000000000000000000, 0.000000000000000000, 0.000000000000000000 ) ) ;
#1489=CARTESIAN_POINT ( 'NONE',  ( -77.56250000204839523, 80.81189881250000440, -10.69163855873948954 ) ) ;
#1493=CARTESIAN_POINT ( 'NONE',  ( -71.93750000409677625, 37.32233047033631124, 17.67766952966369232 ) ) ;
#1496=VECTOR ( 'NONE', #2822, 1000.000000000000000 ) ;
#1501=DIRECTION ( 'NONE',  ( 0.000000000000000000, 0.000000000000000000, 1.000000000000000000 ) ) ;
#1502=CARTESIAN_POINT ( 'NONE',  ( -79.25000000204838102, 80.81189881250001861, -10.69163855873949132 ) ) ;
#1503=DIRECTION ( 'NONE',  ( 0.000000000000000000, 0.000000000000000000, -1.000000000000000000 ) ) ;
#1510=FACE_BOUND ( 'NONE', #8213, .T. ) ;
#1511=CARTESIAN_POINT ( 'NONE',  ( 21.62726510572514727, 76.92664994937649681, 1.832148689196935187 ) ) ;
#1512=CARTESIAN_POINT ( 'NONE',  ( -74.93750000204838102, 65.69163855873948421, -25.81189881250000084 ) ) ;
#1521=VECTOR ( 'NONE', #6899, 1000.000000000000000 ) ;
#1527=ORIENTED_EDGE ( 'NONE', *, *, #9135, .T. ) ;
#1530=CARTESIAN_POINT ( 'NONE',  ( -77.93750000204838102, 65.69163855873948421, -25.81189881250000440 ) ) ;
#1531=ORIENTED_EDGE ( 'NONE', *, *, #9448, .F. ) ;
#1537=DIRECTION ( 'NONE',  ( 0.000000000000000000, 0.000000000000000000, -1.000000000000000000 ) ) ;
#1541=VECTOR ( 'NONE', #8889, 1000.000000000000000 ) ;
#1547=ADVANCED_FACE ( 'NONE', ( #1051 ), #3753, .T. ) ;
#1549=CARTESIAN_POINT ( 'NONE',  ( -75.59375000409679046, 80.00000000000001421, -10.35533905932737753 ) ) ;
#1550=LINE ( 'NONE', #6180, #928 ) ;
#1552=CIRCLE ( 'NONE', #10724, 24.99999999999999645 ) ;
#1558=CARTESIAN_POINT ( 'NONE',  ( -74.00000000000000000, 55.00000000000000000, -24.99999999999999645 ) ) ;
#1560=CARTESIAN_POINT ( 'NONE',  ( 39.99999999999999289, 55.00000000000000000, 0.000000000000000000 ) ) ;
#1562=CARTESIAN_POINT ( 'NONE',  ( -77.93750000204838102, 65.69163855873948421, -25.81189881250000440 ) ) ;
#1570=CARTESIAN_POINT ( 'NONE',  ( -79.43750000204838102, 55.00000000000000000, -25.81189881249999729 ) ) ;
#1571=CARTESIAN_POINT ( 'NONE',  ( -78.50000000000000000, 55.00000000000000000, -24.99999999999999645 ) ) ;
#1572=CARTESIAN_POINT ( 'NONE',  ( 1.476596942546186009, 65.05810802274424987, 19.56659622200108473 ) ) ;
#1576=DIRECTION ( 'NONE',  ( -1.000000000000000000, -0.000000000000000000, -0.000000000000000000 ) ) ;
#1586=CARTESIAN_POINT ( 'NONE',  ( -78.96875000204839523, 73.25176868561975141, 18.25176868561974075 ) ) ;
#1597=LINE ( 'NONE', #9576, #4710 ) ;
#1603=CARTESIAN_POINT ( 'NONE',  ( -72.21875000409676204, 65.35533905932737753, 24.99999999999999645 ) ) ;
#1605=LINE ( 'NONE', #5390, #2905 ) ;
#1609=DIRECTION ( 'NONE',  ( 1.000000000000000000, 0.000000000000000000, 0.000000000000000000 ) ) ;
#1614=CARTESIAN_POINT ( 'NONE',  ( -79.34375000204839523, 73.25176868561975141, -18.25176868561974430 ) ) ;
#1619=ADVANCED_FACE ( 'NONE', ( #8369 ), #2009, .F. ) ;
#1624=CARTESIAN_POINT ( 'NONE',  ( 0.7390892720871951038, 65.01136756371364811, -19.59014205680648502 ) ) ;
#1625=CARTESIAN_POINT ( 'NONE',  ( -74.84375000204839523, 73.25176868561975141, -18.25176868561974430 ) ) ;
#1630=CARTESIAN_POINT ( 'NONE',  ( -15.00000000000000000, -30.00000000000000000, -10.00000000000000000 ) ) ;
#1640=CARTESIAN_POINT ( 'NONE',  ( -75.68750000204838102, 44.30836144126053000, 25.81189881250000795 ) ) ;
#1662=CARTESIAN_POINT ( 'NONE',  ( -71.65625000409677625, 30.00000000000000355, -10.35533905932738108 ) ) ;
#1672=CARTESIAN_POINT ( 'NONE',  ( -77.46875000204839523, 73.25176868561975141, 18.25176868561974075 ) ) ;
#1677=EDGE_LOOP ( 'NONE', ( #5269, #4436, #10694, #736 ) ) ;
#1678=CARTESIAN_POINT ( 'NONE',  ( 10.32208524953959916, 68.72075925444976008, 20.90353566436339960 ) ) ;
#1680=DIRECTION ( 'NONE',  ( 1.000000000000000000, 0.000000000000000000, 0.000000000000000000 ) ) ;
#1681=CARTESIAN_POINT ( 'NONE',  ( -15.00000000000000355, 5.000000000000000000, 30.00000000000000711 ) ) ;
#1683=AXIS2_PLACEMENT_3D ( 'NONE', #7917, #6012, #8752 ) ;
#1691=DIRECTION ( 'NONE',  ( 0.000000000000000000, 1.000000000000000000, 0.000000000000000000 ) ) ;
#1693=EDGE_CURVE ( 'NONE', #8038, #5411, #11291, .T. ) ;
#1704=CARTESIAN_POINT ( 'NONE',  ( -75.12500000204838102, 44.30836144126050158, -25.81189881249999374 ) ) ;
#1705=VECTOR ( 'NONE', #10638, 1000.000000000000000 ) ;
#1709=VERTEX_POINT ( 'NONE', #1175 ) ;
#1711=AXIS2_PLACEMENT_3D ( 'NONE', #5682, #148, #5558 ) ;
#1729=FACE_OUTER_BOUND ( 'NONE', #10500, .T. ) ;
#1735=CARTESIAN_POINT ( 'NONE',  ( -75.68750000204838102, 44.30836144126053000, 25.81189881250000795 ) ) ;
#1738=CARTESIAN_POINT ( 'NONE',  ( -78.31250000204839523, 29.18810118750000981, 10.69163855873950020 ) ) ;
#1739=AXIS2_PLACEMENT_3D ( 'NONE', #8826, #718, #6918 ) ;
#1747=VERTEX_POINT ( 'NONE', #454 ) ;
#1754=CARTESIAN_POINT ( 'NONE',  ( -13.89602465295604539, 70.84623132619663011, -15.29986294999528695 ) ) ;
#1760=CARTESIAN_POINT ( 'NONE',  ( -76.25000000204838102, 65.69163855873948421, -25.81189881250000440 ) ) ;
#1774=DIRECTION ( 'NONE',  ( -1.000000000000000000, -0.000000000000000000, -0.000000000000000000 ) ) ;
#1781=CARTESIAN_POINT ( 'NONE',  ( -77.75000000000000000, 55.00000000000000000, 24.99999999999999645 ) ) ;
#1788=CARTESIAN_POINT ( 'NONE',  ( -72.21875000204838102, 36.74823131438024859, -18.25176868561973720 ) ) ;
#1793=CARTESIAN_POINT ( 'NONE',  ( -1.625240267017640655E-20, 65.42943686846950868, 22.72062601704910634 ) ) ;
#1796=CARTESIAN_POINT ( 'NONE',  ( -77.28125000409677625, 65.35533905932743437, -24.99999999999994671 ) ) ;
#1797=CARTESIAN_POINT ( 'NONE',  ( -77.84374999999997158, 65.35533905932209109, 25.00000000000518341 ) ) ;
#1802=( BOUNDED_CURVE ( )  B_SPLINE_CURVE ( 2, ( #6603, #10230, #3115, #523, #6781, #10464, #5149, #4975, #3286, #1374, #6000, #4184, #5037, #2208, #2264, #10410, #5877, #8683, #8801, #1489, #580, #9634, #4246, #5937, #466, #4123, #1429, #11361, #10580, #7906, #8626, #6955, #6838, #9692, #9517, #7786, #5092, #2381, #6056, #11535, #6894, #11415, #1309, #408, #7670, #11305, #4073, #7730, #7846, #9578, #3170, #3226, #10522, #2330, #8740, #11474, #7531, #384, #8359, #8607, #261, #3029, #6697, #11098, #6515, #3804, #2913, #6759, #4765, #2125, #1041, #10267, #2065, #3092, #5736, #1284, #8421, #11279, #10328, #205, #9253, #2182, #8485, #5799, #4707, #5853, #8540 ),
 .UNSPECIFIED., .F., .T. ) 
 B_SPLINE_CURVE_WITH_KNOTS ( ( 3, 2, 2, 2, 2, 2, 2, 2, 2, 2, 2, 2, 2, 2, 2, 2, 2, 2, 2, 2, 2, 2, 2, 2, 2, 2, 2, 2, 2, 2, 2, 2, 2, 2, 2, 2, 2, 2, 2, 2, 2, 2, 2, 3 ),
 ( 0.000000000000000000, 0.02083333333333333218, 0.04166666666666666435, 0.06250000000000000000, 0.08333333333333332871, 0.1041666666666666713, 0.1250000000000000000, 0.1458333333333333148, 0.1666666666666666574, 0.1874999999999999722, 0.2083333333333333426, 0.2291666666666666852, 0.2500000000000000000, 0.2708333333333333148, 0.2916666666666666297, 0.3125000000000000000, 0.3333333333333333148, 0.3541666666666666852, 0.3749999999999999445, 0.3958333333333333148, 0.4166666666666666852, 0.4375000000000000000, 0.4583333333333333703, 0.4791666666666666852, 0.5000000000000000000, 0.5208333333333333703, 0.5416666666666666297, 0.5625000000000000000, 0.5833333333333332593, 0.6041666666666666297, 0.6250000000000000000, 0.6458333333333333703, 0.6666666666666666297, 0.6875000000000000000, 0.7083333333333333703, 0.7291666666666666297, 0.7499999999999998890, 0.7708333333333333703, 0.7916666666666666297, 0.8125000000000000000, 0.8333333333333333703, 0.8541666666666666297, 0.8750000000000000000, 0.8888490476107191451 ),
 .UNSPECIFIED. ) 
 CURVE ( )  GEOMETRIC_REPRESENTATION_ITEM ( )  RATIONAL_B_SPLINE_CURVE ( ( 1.000000000000000000, 0.9238795325112867385, 1.000000000000000000, 0.9238795325112867385, 1.000000000000000000, 0.9238795325112867385, 1.000000000000000000, 0.9238795325112867385, 1.000000000000000000, 0.9238795325112867385, 1.000000000000000000, 0.9238795325112867385, 1.000000000000000000, 0.9238795325112867385, 1.000000000000000000, 0.9238795325112867385, 1.000000000000000000, 0.9238795325112867385, 1.000000000000000000, 0.9238795325112867385, 1.000000000000000000, 0.9238795325112867385, 1.000000000000000000, 0.9238795325112867385, 1.000000000000000000, 0.9238795325112867385, 1.000000000000000000, 0.9238795325112867385, 1.000000000000000000, 0.9238795325112867385, 1.000000000000000000, 0.9238795325112867385, 1.000000000000000000, 0.9238795325112867385, 1.000000000000000000, 0.9238795325112867385, 1.000000000000000000, 0.9238795325112867385, 1.000000000000000000, 0.9238795325112867385, 1.000000000000000000, 0.9238795325112867385, 1.000000000000000000, 0.9238795325112867385, 1.000000000000000000, 0.9238795325112867385, 1.000000000000000000, 0.9238795325112867385, 1.000000000000000000, 0.9238795325112867385, 1.000000000000000000, 0.9238795325112867385, 1.000000000000000000, 0.9238795325112867385, 1.000000000000000000, 0.9238795325112867385, 1.000000000000000000, 0.9238795325112867385, 1.000000000000000000, 0.9238795325112867385, 1.000000000000000000, 0.9238795325112867385, 1.000000000000000000, 0.9238795325112867385, 1.000000000000000000, 0.9238795325112867385, 1.000000000000000000, 0.9238795325112867385, 1.000000000000000000, 0.9238795325112867385, 1.000000000000000000, 0.9238795325112867385, 1.000000000000000000, 0.9238795325112867385, 1.000000000000000000, 0.9238795325112867385, 1.000000000000000000, 0.9238795325112867385, 1.000000000000000000, 0.9238795325112867385, 1.000000000000000000, 0.9238795325112867385, 1.000000000000000000, 0.9238795325112867385, 1.000000000000000000, 0.9493985930367334625, 0.9660721903170175207 ) ) 
 REPRESENTATION_ITEM ( '' )  );
#1805=CARTESIAN_POINT ( 'NONE',  ( -12.86143404212990227, 70.11511422732331766, -16.01369128662254582 ) ) ;
#1812=CARTESIAN_POINT ( 'NONE',  ( -74.00000000204839523, 29.18810118750000981, 10.69163855873950020 ) ) ;
#1813=ORIENTED_EDGE ( 'NONE', *, *, #2839, .T. ) ;
#1832=CARTESIAN_POINT ( 'NONE',  ( -76.90625000000005684, 65.35533905932732068, -24.99999999999990052 ) ) ;
#1837=PRODUCT_DEFINITION_SHAPE ( 'NONE', 'NONE',  #133 ) ;
#1845=CARTESIAN_POINT ( 'NONE',  ( -10.31596542140328587, 68.71721060802151726, -20.90586008767603587 ) ) ;
#1849=CARTESIAN_POINT ( 'NONE',  ( -79.25000000204838102, 65.69163855873948421, -25.81189881250000440 ) ) ;
#1856=DIRECTION ( 'NONE',  ( -0.000000000000000000, -1.000000000000000000, -0.000000000000000000 ) ) ;
#1860=LINE ( 'NONE', #9232, #10684 ) ;
#1866=CARTESIAN_POINT ( 'NONE',  ( -20.07101753429484248, 75.63268020737004349, 7.663897408568258740 ) ) ;
#1869=CARTESIAN_POINT ( 'NONE',  ( -74.00000000000000000, 55.00000000000000000, -24.99999999999999645 ) ) ;
#1870=EDGE_LOOP ( 'NONE', ( #218, #5857, #11767, #5435 ) ) ;
#1873=CARTESIAN_POINT ( 'NONE',  ( -77.84375000204839523, 55.00000000000000000, -25.81189881249999729 ) ) ;
#1879=VERTEX_POINT ( 'NONE', #99 ) ;
#1881=EDGE_CURVE ( 'NONE', #494, #7502, #39, .T. ) ;
#1888=CARTESIAN_POINT ( 'NONE',  ( -79.43750000204838102, 55.00000000000000000, -25.81189881249999729 ) ) ;
#1893=CARTESIAN_POINT ( 'NONE',  ( -71.37500000409677625, 55.00000000000000000, -24.99999999999999645 ) ) ;
#1899=CARTESIAN_POINT ( 'NONE',  ( -78.12500000409677625, 55.00000000000000000, 24.99999999999999645 ) ) ;
#1902=CARTESIAN_POINT ( 'NONE',  ( -72.78125000204838102, 55.00000000000000000, 25.81189881249999729 ) ) ;
#1906=CARTESIAN_POINT ( 'NONE',  ( -23.32960838815753490, 78.33373921288500696, -8.983038135490025056 ) ) ;
#1910=CARTESIAN_POINT ( 'NONE',  ( -78.40625000204839523, 36.74823131438026280, 18.25176868561974786 ) ) ;
#1916=CARTESIAN_POINT ( 'NONE',  ( 36.99999999999999289, 55.00000000000000000, 0.000000000000000000 ) ) ;
#1921=AXIS2_PLACEMENT_3D ( 'NONE', #8467, #1141, #6679 ) ;
#1922=CARTESIAN_POINT ( 'NONE',  ( -74.28125000000007105, 30.00000000000014211, -10.35533905932732601 ) ) ;
#1928=CARTESIAN_POINT ( 'NONE',  ( -5.007765583651338837, 65.88190602726542977, -19.12178772468223897 ) ) ;
#1933=CARTESIAN_POINT ( 'NONE',  ( -73.90625000409680467, 80.00000000000001421, 10.35533905932737397 ) ) ;
#1934=ORIENTED_EDGE ( 'NONE', *, *, #4687, .F. ) ;
#1936=CARTESIAN_POINT ( 'NONE',  ( -78.31250000204839523, 29.18810118750000981, 10.69163855873950020 ) ) ;
#1942=CLOSED_SHELL ( 'NONE', ( #6086, #7241, #2159, #1410, #1619, #9768, #5316, #10444, #2047, #4900, #1547, #8436, #6698, #948, #7896, #1337, #6978, #427, #5335, #5578, #73, #2882, #9885, #3822, #4820, #11851, #437, #1225, #5185, #3966, #9168, #2788, #11339, #4188, #5295, #7143, #5894, #1146, #7469, #2200, #9443, #10633, #7710, #4333, #10036, #6330 ) ) ;
#1946=CARTESIAN_POINT ( 'NONE',  ( -72.68750000409677625, 72.67766952966368876, -17.67766952966368876 ) ) ;
#1951=CARTESIAN_POINT ( 'NONE',  ( -72.87500000409677625, 55.00000000000000000, -24.99999999999999645 ) ) ;
#1959=EDGE_CURVE ( 'NONE', #9573, #11173, #10525, .T. ) ;
#1961=CARTESIAN_POINT ( 'NONE',  ( -78.31250000409679046, 72.67766952966368876, 17.67766952966368521 ) ) ;
#1963=ORIENTED_EDGE ( 'NONE', *, *, #3528, .T. ) ;
#1968=CARTESIAN_POINT ( 'NONE',  ( -73.81250000204839523, 29.18810118750000626, -10.69163855873949309 ) ) ;
#1971=FACE_OUTER_BOUND ( 'NONE', #1220, .T. ) ;
#1973=CARTESIAN_POINT ( 'NONE',  ( -15.00000000000000355, 5.000000000000000000, 30.00000000000000711 ) ) ;
#1975=PLANE ( 'NONE',  #3660 ) ;
#1979=CARTESIAN_POINT ( 'NONE',  ( -80.00000000000000000, 55.00000000000000000, -24.99999999999999645 ) ) ;
#1995=CARTESIAN_POINT ( 'NONE',  ( -73.43750000204839523, 65.69163855873948421, -25.81189881250000440 ) ) ;
#1996=CARTESIAN_POINT ( 'NONE',  ( 39.99999999999999289, 55.00000000000000000, 24.99999999999999645 ) ) ;
#2007=DIRECTION ( 'NONE',  ( -0.000000000000000000, -1.000000000000000000, -0.000000000000000000 ) ) ;
#2009=CYLINDRICAL_SURFACE ( 'NONE', #1711, 22.00000000000000000 ) ;
#2019=EDGE_LOOP ( 'NONE', ( #5337, #2089, #3376, #6161 ) ) ;
#2025=CARTESIAN_POINT ( 'NONE',  ( -17.84886775434581452, 73.89817018583475772, -16.37880432067737146 ) ) ;
#2028=CARTESIAN_POINT ( 'NONE',  ( -73.43750000204839523, 44.30836144126050158, -25.81189881249999374 ) ) ;
#2030=CARTESIAN_POINT ( 'NONE',  ( 14.93568603768559200, 71.73165937744515475, -18.58548037958608390 ) ) ;
#2035=DIRECTION ( 'NONE',  ( -1.000000000000000000, -0.000000000000000000, -0.000000000000000000 ) ) ;
#2036=CARTESIAN_POINT ( 'NONE',  ( -15.00000000000000355, 0.000000000000000000, 30.00000000000000711 ) ) ;
#2040=CARTESIAN_POINT ( 'NONE',  ( -78.68750000000001421, 37.32233047033631124, -17.67766952966368166 ) ) ;
#2046=CARTESIAN_POINT ( 'NONE',  ( -16.77618538223333289, 72.99562347272558327, 12.71320776128724539 ) ) ;
#2047=ADVANCED_FACE ( 'NONE', ( #11062 ), #4730, .T. ) ;
#2051=ORIENTED_EDGE ( 'NONE', *, *, #7567, .T. ) ;
#2053=CARTESIAN_POINT ( 'NONE',  ( -74.28125000409677625, 65.35533905932754806, -24.99999999999982947 ) ) ;
#2054=VERTEX_POINT ( 'NONE', #942 ) ;
#2064=ORIENTED_EDGE ( 'NONE', *, *, #10321, .F. ) ;
#2065=CARTESIAN_POINT ( 'NONE',  ( -72.59375000204838102, 55.00000000000000000, 25.81189881249999729 ) ) ;
#2066=CARTESIAN_POINT ( 'NONE',  ( -72.87500000409677625, 55.00000000000000000, -24.99999999999999645 ) ) ;
#2068=ORIENTED_EDGE ( 'NONE', *, *, #7447, .F. ) ;
#2073=DIRECTION ( 'NONE',  ( 1.000000000000000000, 0.000000000000000000, 0.000000000000000000 ) ) ;
#2074=ORIENTED_EDGE ( 'NONE', *, *, #4284, .T. ) ;
#2084=LINE ( 'NONE', #9744, #9868 ) ;
#2089=ORIENTED_EDGE ( 'NONE', *, *, #6623, .T. ) ;
#2090=CARTESIAN_POINT ( 'NONE',  ( -73.34375000204839523, 55.00000000000000000, -25.81189881249999729 ) ) ;
#2091=CONICAL_SURFACE ( 'NONE', #8793, 20.00000000000000000, 0.1745329251994333364 ) ;
#2092=CARTESIAN_POINT ( 'NONE',  ( 14.99999999999999645, 0.000000000000000000, -29.99999999999999289 ) ) ;
#2093=CARTESIAN_POINT ( 'NONE',  ( 1.711474602913919396, 65.50696799861361797, -22.68545269630726224 ) ) ;
#2108=CARTESIAN_POINT ( 'NONE',  ( -72.78125000000008527, 30.00000000000014566, -10.35533905932732424 ) ) ;
#2109=CARTESIAN_POINT ( 'NONE',  ( 39.99999999999999289, 55.00000000000000000, 0.000000000000000000 ) ) ;
#2117=CARTESIAN_POINT ( 'NONE',  ( -75.31250000204839523, 29.18810118750000981, 10.69163855873950020 ) ) ;
#2119=CARTESIAN_POINT ( 'NONE',  ( -79.34375000000000000, 65.35533905932734910, 24.99999999999997158 ) ) ;
#2121=VECTOR ( 'NONE', #4741, 1000.000000000000000 ) ;
#2123=CARTESIAN_POINT ( 'NONE',  ( -78.12500000409677625, 55.00000000000000000, 24.99999999999999645 ) ) ;
#2125=CARTESIAN_POINT ( 'NONE',  ( -72.87500000204839523, 80.81189881250000440, 10.69163855873948243 ) ) ;
#2142=CIRCLE ( 'NONE', #8635, 22.00000000000000000 ) ;
#2144=DIRECTION ( 'NONE',  ( -1.000000000000000000, 0.000000000000000000, 0.000000000000000000 ) ) ;
#2151=CARTESIAN_POINT ( 'NONE',  ( -14.31771318061109532, 71.29407831320283151, 18.96900533006995104 ) ) ;
#2154=CARTESIAN_POINT ( 'NONE',  ( -72.12500000204840944, 29.18810118750000626, -10.69163855873949309 ) ) ;
#2156=CARTESIAN_POINT ( 'NONE',  ( 25.27762860081886487, 79.98954112471153621, -0.8412697711426854186 ) ) ;
#2159=ADVANCED_FACE ( 'NONE', ( #208 ), #6725, .F. ) ;
#2163=CARTESIAN_POINT ( 'NONE',  ( -75.96875000000000000, 30.00000000000001421, 10.35533905932739174 ) ) ;
#2168=CARTESIAN_POINT ( 'NONE',  ( -17.79883679810149744, 73.80018128902068497, 11.43000178191448235 ) ) ;
#2173=CARTESIAN_POINT ( 'NONE',  ( -76.81250000204838102, 29.18810118750000626, -10.69163855873949132 ) ) ;
#2177=CARTESIAN_POINT ( 'NONE',  ( -74.09375000204839523, 55.00000000000000000, 25.81189881249999729 ) ) ;
#2178=FACE_OUTER_BOUND ( 'NONE', #3367, .T. ) ;
#2182=CARTESIAN_POINT ( 'NONE',  ( -71.75000000204840944, 65.69163855873948421, -25.81189881250000084 ) ) ;
#2184=DIRECTION ( 'NONE',  ( -1.000000000000000000, -0.000000000000000000, -0.000000000000000000 ) ) ;
#2189=LINE ( 'NONE', #5079, #10498 ) ;
#2194=PLANE ( 'NONE',  #7492 ) ;
#2200=ADVANCED_FACE ( 'NONE', ( #6212 ), #907, .T. ) ;
#2208=CARTESIAN_POINT ( 'NONE',  ( -78.12500000204839523, 29.18810118750000626, -10.69163855873949132 ) ) ;
#2209=DIRECTION ( 'NONE',  ( 1.000000000000000000, 0.000000000000000000, 0.000000000000000000 ) ) ;
#2214=CARTESIAN_POINT ( 'NONE',  ( -72.96875000204838102, 80.81189881250000440, -1.580522963032174394E-15 ) ) ;
#2220=CARTESIAN_POINT ( 'NONE',  ( -15.00000000000000000, 39.99999999999999289, -20.00000000000000000 ) ) ;
#2223=CARTESIAN_POINT ( 'NONE',  ( -73.90625000000001421, 65.35533905932737753, -24.99999999999999645 ) ) ;
#2233=CARTESIAN_POINT ( 'NONE',  ( -76.06250000204839523, 80.81189881250000440, 10.69163855873948243 ) ) ;
#2234=EDGE_LOOP ( 'NONE', ( #4086, #9591, #2051, #5911, #3105, #4250, #5327, #8599 ) ) ;
#2242=DIRECTION ( 'NONE',  ( 0.000000000000000000, 1.000000000000000000, 0.000000000000000000 ) ) ;
#2260=EDGE_LOOP ( 'NONE', ( #6399, #160, #887, #11432 ) ) ;
#2262=DIRECTION ( 'NONE',  ( 0.000000000000000000, -1.000000000000000000, 0.000000000000000000 ) ) ;
#2264=CARTESIAN_POINT ( 'NONE',  ( -78.03125000204839523, 36.74823131438024859, -18.25176868561973720 ) ) ;
#2265=DIRECTION ( 'NONE',  ( 0.000000000000000000, 0.000000000000000000, -1.000000000000000000 ) ) ;
#2268=CARTESIAN_POINT ( 'NONE',  ( -77.46875000409679046, 44.64466094067260826, -24.99999999999998934 ) ) ;
#2269=CARTESIAN_POINT ( 'NONE',  ( -80.00000000000000000, 55.00000000000000000, -24.99999999999999645 ) ) ;
#2271=SURFACE_STYLE_USAGE ( .BOTH. , #9026 ) ;
#2278=ORIENTED_EDGE ( 'NONE', *, *, #4024, .T. ) ;
#2282=CARTESIAN_POINT ( 'NONE',  ( -78.03124999999998579, 80.00000000000001421, 10.35533905932737397 ) ) ;
#2284=AXIS2_PLACEMENT_3D ( 'NONE', #10192, #10528, #120 ) ;
#2290=DIRECTION ( 'NONE',  ( 0.000000000000000000, 0.000000000000000000, 1.000000000000000000 ) ) ;
#2295=CARTESIAN_POINT ( 'NONE',  ( 20.34144692743802807, 75.85564821147012537, -7.037142918007486259 ) ) ;
#2298=CARTESIAN_POINT ( 'NONE',  ( -72.21875000204838102, 29.18810118750000271, 4.741568889096522788E-15 ) ) ;
#2311=CARTESIAN_POINT ( 'NONE',  ( 39.99999999999999289, 55.00000000000000000, 0.000000000000000000 ) ) ;
#2314=CONICAL_SURFACE ( 'NONE', #969, 20.00000000000000000, 0.1745329251994333364 ) ;
#2317=LINE ( 'NONE', #3107, #6259 ) ;
#2318=( BOUNDED_CURVE ( )  B_SPLINE_CURVE ( 2, ( #2570, #7016, #10587, #2387, #9867, #1662, #586, #4253, #10639 ),
 .UNSPECIFIED., .F., .T. ) 
 B_SPLINE_CURVE_WITH_KNOTS ( ( 3, 2, 2, 2, 3 ),
 ( 0.7500000000000006661, 0.7708333333333340365, 0.7916666666666672958, 0.8125000000000006661, 0.8333333333333340365 ),
 .UNSPECIFIED. ) 
 CURVE ( )  GEOMETRIC_REPRESENTATION_ITEM ( )  RATIONAL_B_SPLINE_CURVE ( ( 0.9999999999999975575, 0.9238795325112891810, 1.000000000000000000, 0.9238795325112867385, 1.000000000000000000, 0.9238795325112867385, 1.000000000000000000, 0.9238795325112842960, 1.000000000000002442 ) ) 
 REPRESENTATION_ITEM ( '' )  );
#2326=EDGE_CURVE ( 'NONE', #8979, #10562, #10255, .T. ) ;
#2330=CARTESIAN_POINT ( 'NONE',  ( -74.37500000204838102, 80.81189881250000440, 10.69163855873948243 ) ) ;
#2331=CARTESIAN_POINT ( 'NONE',  ( -4.228830400747147777, 66.03037594905248397, 22.43534422001513207 ) ) ;
#2333=ORIENTED_EDGE ( 'NONE', *, *, #3649, .F. ) ;
#2335=CARTESIAN_POINT ( 'NONE',  ( -72.40625000409677625, 80.00000000000001421, 10.35533905932737397 ) ) ;
#2344=VERTEX_POINT ( 'NONE', #1869 ) ;
#2345=DIRECTION ( 'NONE',  ( -0.000000000000000000, -1.000000000000000000, -0.000000000000000000 ) ) ;
#2346=CARTESIAN_POINT ( 'NONE',  ( -75.12500000000000000, 80.00000000000000000, -1.530808498934191324E-15 ) ) ;
#2347=FACE_OUTER_BOUND ( 'NONE', #7174, .T. ) ;
#2354=CARTESIAN_POINT ( 'NONE',  ( 21.71450277048158739, 76.99996143417730821, 0.3671359477368970614 ) ) ;
#2355=CARTESIAN_POINT ( 'NONE',  ( -76.15625000204838102, 80.81189881250000440, -1.580522963032174394E-15 ) ) ;
#2356=ORIENTED_EDGE ( 'NONE', *, *, #6842, .F. ) ;
#2362=EDGE_CURVE ( 'NONE', #4746, #1747, #6389, .T. ) ;
#2369=DIRECTION ( 'NONE',  ( -0.000000000000000000, -1.000000000000000000, -0.000000000000000000 ) ) ;
#2371=EDGE_LOOP ( 'NONE', ( #10304, #5274 ) ) ;
#2381=CARTESIAN_POINT ( 'NONE',  ( -75.87500000204838102, 80.81189881250000440, 10.69163855873948243 ) ) ;
#2385=CARTESIAN_POINT ( 'NONE',  ( -74.75000000409677625, 30.00000000000000355, 4.592425496802573578E-15 ) ) ;
#2387=CARTESIAN_POINT ( 'NONE',  ( -71.84375000409677625, 30.00000000000001421, 10.35533905932739174 ) ) ;
#2392=EDGE_CURVE ( 'NONE', #10874, #8848, #5605, .T. ) ;
#2396=CARTESIAN_POINT ( 'NONE',  ( 6.123233995736766282E-16, -30.00000000000000000, 5.000000000000000000 ) ) ;
#2398=CARTESIAN_POINT ( 'NONE',  ( -72.96875000000000000, 30.00000000000001421, 10.35533905932739174 ) ) ;
#2401=CARTESIAN_POINT ( 'NONE',  ( 36.99999999999999289, 55.00000000000000000, 0.000000000000000000 ) ) ;
#2408=CARTESIAN_POINT ( 'NONE',  ( 12.85511924628072755, 70.12525320288015962, 15.98407836417939443 ) ) ;
#2414=DIRECTION ( 'NONE',  ( 0.000000000000000000, 0.000000000000000000, 1.000000000000000000 ) ) ;
#2430=CARTESIAN_POINT ( 'NONE',  ( -76.90625000204838102, 29.18810118750000271, 4.741568889096522788E-15 ) ) ;
#2433=ORIENTED_EDGE ( 'NONE', *, *, #11406, .T. ) ;
#2446=LINE ( 'NONE', #8084, #6790 ) ;
#2449=ORIENTED_EDGE ( 'NONE', *, *, #10815, .F. ) ;
#2450=CARTESIAN_POINT ( 'NONE',  ( -74.65625000409679046, 30.00000000000000355, -10.35533905932738108 ) ) ;
#2457=CARTESIAN_POINT ( 'NONE',  ( 36.99999999999999289, 55.00000000000000000, 0.000000000000000000 ) ) ;
#2461=CARTESIAN_POINT ( 'NONE',  ( -72.12500000000000000, 80.00000000000000000, -1.530808498934191324E-15 ) ) ;
#2465=PRODUCT_DEFINITION_CONTEXT ( 'detailed design', #5550, 'design' ) ;
#2472=CARTESIAN_POINT ( 'NONE',  ( 7.639074212767907213, 67.00087384642168331, -18.44261089144852050 ) ) ;
#2474=CARTESIAN_POINT ( 'NONE',  ( -74.37500000204838102, 65.69163855873949842, 25.81189881250000084 ) ) ;
#2478=CARTESIAN_POINT ( 'NONE',  ( 9.999999999999994671, -24.99999999999999645, -10.00000000000000000 ) ) ;
#2493=CARTESIAN_POINT ( 'NONE',  ( -76.81250000204838102, 29.18810118750000626, -10.69163855873949309 ) ) ;
#2496=( BOUNDED_CURVE ( )  B_SPLINE_CURVE ( 2, ( #2534, #2593, #2767, #10059, #10903, #51, #8945, #1797, #3492 ),
 .UNSPECIFIED., .F., .T. ) 
 B_SPLINE_CURVE_WITH_KNOTS ( ( 3, 2, 2, 2, 3 ),
 ( 0.1584082455038353654, 0.1782132311131151281, 0.1980182167223948908, 0.2178232023316745980, 0.2376281879409543607 ),
 .UNSPECIFIED. ) 
 CURVE ( )  GEOMETRIC_REPRESENTATION_ITEM ( )  RATIONAL_B_SPLINE_CURVE ( ( 1.000000000000020650, 0.9238795325112661994, 1.000000000000000000, 0.9238795325112868495, 1.000000000000000000, 0.9238795325112868495, 1.000000000000000000, 0.9238795325112363344, 1.000000000000050404 ) ) 
 REPRESENTATION_ITEM ( '' )  );
#2499=SHAPE_REPRESENTATION_RELATIONSHIP ( 'NONE' , 'NONE' ,  #423, #9980 ) ;
#2509=PLANE ( 'NONE',  #7169 ) ;
#2515=CARTESIAN_POINT ( 'NONE',  ( -71.65625000409677625, 30.00000000000000355, -10.35533905932738108 ) ) ;
#2516=LINE ( 'NONE', #5154, #5165 ) ;
#2519=ORIENTED_EDGE ( 'NONE', *, *, #426, .T. ) ;
#2521=EDGE_CURVE ( 'NONE', #7145, #10896, #5093, .T. ) ;
#2526=CARTESIAN_POINT ( 'NONE',  ( -76.25000000204838102, 80.81189881250001861, -10.69163855873949132 ) ) ;
#2533=CARTESIAN_POINT ( 'NONE',  ( -78.87500000000002842, 30.00000000000003553, 4.592425496802568845E-15 ) ) ;
#2534=CARTESIAN_POINT ( 'NONE',  ( -78.50000000000000000, 55.00000000000000000, -24.99999999999999645 ) ) ;
#2535=CARTESIAN_POINT ( 'NONE',  ( -71.84375000204838102, 73.25176868561975141, -18.25176868561974430 ) ) ;
#2540=LINE ( 'NONE', #787, #10162 ) ;
#2551=ORIENTED_EDGE ( 'NONE', *, *, #7785, .T. ) ;
#2552=CARTESIAN_POINT ( 'NONE',  ( 0.000000000000000000, 110.0000000000000000, 0.000000000000000000 ) ) ;
#2567=ORIENTED_EDGE ( 'NONE', *, *, #3528, .F. ) ;
#2568=CARTESIAN_POINT ( 'NONE',  ( -71.75000000409677625, 30.00000000000000355, 4.592425496802573578E-15 ) ) ;
#2570=CARTESIAN_POINT ( 'NONE',  ( -72.12500000409677625, 55.00000000000000000, 24.99999999999999645 ) ) ;
#2575=VERTEX_POINT ( 'NONE', #7101 ) ;
#2577=LINE ( 'NONE', #707, #115 ) ;
#2580=EDGE_CURVE ( 'NONE', #6077, #2686, #10144, .T. ) ;
#2583=CARTESIAN_POINT ( 'NONE',  ( -79.43750000204838102, 65.69163855873948421, -25.81189881250000440 ) ) ;
#2586=EDGE_CURVE ( 'NONE', #10642, #9073, #399, .T. ) ;
#2589=CARTESIAN_POINT ( 'NONE',  ( 19.98279345720612454, 75.57879140538503293, 14.21315688551485579 ) ) ;
#2593=CARTESIAN_POINT ( 'NONE',  ( -78.40625000000005684, 65.35533905932518906, -25.00000000000207478 ) ) ;
#2594=CARTESIAN_POINT ( 'NONE',  ( -73.62500000204838102, 44.30836144126049447, -25.81189881249999019 ) ) ;
#2595=VERTEX_POINT ( 'NONE', #11238 ) ;
#2597=LINE ( 'NONE', #5241, #1541 ) ;
#2602=VECTOR ( 'NONE', #5265, 1000.000000000000000 ) ;
#2608=CARTESIAN_POINT ( 'NONE',  ( -75.59375000204839523, 36.74823131438026280, 18.25176868561974786 ) ) ;
#2609=CONICAL_SURFACE ( 'NONE', #7769, 17.04557674096337649, 0.1745329251994333364 ) ;
#2621=DIRECTION ( 'NONE',  ( 0.000000000000000000, 0.9848077530122080203, 0.1736481776669307198 ) ) ;
#2632=CARTESIAN_POINT ( 'NONE',  ( -74.84375000000005684, 65.35533905932891230, 24.99999999999828404 ) ) ;
#2635=( BOUNDED_CURVE ( )  B_SPLINE_CURVE ( 2, ( #815, #1832, #4598, #10938, #5444, #7190, #756, #4485, #9208 ),
 .UNSPECIFIED., .F., .T. ) 
 B_SPLINE_CURVE_WITH_KNOTS ( ( 3, 2, 2, 2, 3 ),
 ( 0.3168733201082642448, 0.3366713418703649596, 0.3564693636324655635, 0.3762673853945661673, 0.3960654071566668821 ),
 .UNSPECIFIED. ) 
 CURVE ( )  GEOMETRIC_REPRESENTATION_ITEM ( )  RATIONAL_B_SPLINE_CURVE ( ( 1.000000000000000000, 0.9238795325112868495, 1.000000000000000000, 0.9238795325112868495, 1.000000000000000000, 0.9238795325112868495, 1.000000000000000000, 0.9238795325112868495, 1.000000000000000000 ) ) 
 REPRESENTATION_ITEM ( '' )  );
#2638=CARTESIAN_POINT ( 'NONE',  ( -74.56250000204839523, 80.81189881250001861, 10.69163855873948599 ) ) ;
#2642=CARTESIAN_POINT ( 'NONE',  ( -76.90625000204839523, 36.74823131438026280, 18.25176868561974786 ) ) ;
#2651=CARTESIAN_POINT ( 'NONE',  ( -73.34375000204839523, 73.25176868561975141, -18.25176868561974430 ) ) ;
#2652=EDGE_LOOP ( 'NONE', ( #9846, #6577, #4030, #3111 ) ) ;
#2653=CYLINDRICAL_SURFACE ( 'NONE', #3545, 24.99999999999999645 ) ;
#2657=B_SPLINE_CURVE_WITH_KNOTS ( 'NONE', 3,
 ( #9833, #4390, #5057, #661 ),
 .UNSPECIFIED., .F., .F.,
 ( 4, 4 ),
 ( 0.000000000000000000, 1.000000000000000000 ),
 .UNSPECIFIED. ) ;
#2661=CARTESIAN_POINT ( 'NONE',  ( -17.98788677490622234, 73.94881694393184546, -11.19406059795755226 ) ) ;
#2668=CARTESIAN_POINT ( 'NONE',  ( -77.09375000204839523, 36.74823131438026280, 18.25176868561974786 ) ) ;
#2686=VERTEX_POINT ( 'NONE', #3947 ) ;
#2701=CARTESIAN_POINT ( 'NONE',  ( -74.09375000204839523, 36.74823131438026280, 18.25176868561974786 ) ) ;
#2703=ORIENTED_EDGE ( 'NONE', *, *, #9671, .T. ) ;
#2704=CARTESIAN_POINT ( 'NONE',  ( -75.40625000204839523, 36.74823131438026280, 18.25176868561974786 ) ) ;
#2706=CIRCLE ( 'NONE', #10913, 24.99999999999999645 ) ;
#2712=( BOUNDED_CURVE ( )  B_SPLINE_CURVE ( 2, ( #9519, #8628, #10465, #3171, #6839, #11536, #5385, #9035, #812 ),
 .UNSPECIFIED., .F., .T. ) 
 B_SPLINE_CURVE_WITH_KNOTS ( ( 3, 2, 2, 2, 3 ),
 ( 0.3960654071566668821, 0.4158759072859738448, 0.4356864074152808075, 0.4554969075445878257, 0.4753074076738947884 ),
 .UNSPECIFIED. ) 
 CURVE ( )  GEOMETRIC_REPRESENTATION_ITEM ( )  RATIONAL_B_SPLINE_CURVE ( ( 1.000000000000000000, 0.9238795325112867385, 1.000000000000000000, 0.9238795325112867385, 1.000000000000000000, 0.9238795325112867385, 1.000000000000000000, 0.9238795325112889589, 0.9999999999999977796 ) ) 
 REPRESENTATION_ITEM ( '' )  );
#2723=EDGE_CURVE ( 'NONE', #1879, #7325, #6538, .T. ) ;
#2724=CARTESIAN_POINT ( 'NONE',  ( -21.66281002447331261, 76.95651461112846903, 1.430698443491871474 ) ) ;
#2732=CARTESIAN_POINT ( 'NONE',  ( -73.62500000204839523, 44.30836144126050158, -25.81189881249999374 ) ) ;
#2743=CARTESIAN_POINT ( 'NONE',  ( 14.99999999999999645, 55.00000000000000000, -20.00000000000000000 ) ) ;
#2751=CARTESIAN_POINT ( 'NONE',  ( -77.65624999999998579, 44.64466094066740709, 24.99999999999465672 ) ) ;
#2753=EDGE_LOOP ( 'NONE', ( #1012, #5577 ) ) ;
#2757=CARTESIAN_POINT ( 'NONE',  ( -4.655134714661222084, 66.15614397521940759, -22.37326029429084429 ) ) ;
#2760=CARTESIAN_POINT ( 'NONE',  ( -77.28125000204839523, 73.25176868561975141, 18.25176868561974075 ) ) ;
#2762=CARTESIAN_POINT ( 'NONE',  ( 14.96838742389068244, 71.73858167410611486, 18.60395740379449947 ) ) ;
#2767=CARTESIAN_POINT ( 'NONE',  ( -78.31250000000004263, 72.67766952966363192, -17.67766952966363903 ) ) ;
#2769=DIRECTION ( 'NONE',  ( -0.000000000000000000, -0.000000000000000000, -1.000000000000000000 ) ) ;
#2776=CARTESIAN_POINT ( 'NONE',  ( -1.462190304540868846, 65.05665727266017484, -19.56733247748169191 ) ) ;
#2777=LINE ( 'NONE', #10068, #5506 ) ;
#2782=CARTESIAN_POINT ( 'NONE',  ( -71.53052368722832455, 77.35376350879521112, 12.90594348738575903 ) ) ;
#2788=ADVANCED_FACE ( 'NONE', ( #10228 ), #2609, .F. ) ;
#2806=CARTESIAN_POINT ( 'NONE',  ( 0.000000000000000000, 110.0000000000000000, 30.57961884250791940 ) ) ;
#2811=CARTESIAN_POINT ( 'NONE',  ( -22.24878634527607346, 77.42810750878007298, -11.15476345160014660 ) ) ;
#2815=CARTESIAN_POINT ( 'NONE',  ( -78.03125000204839523, 36.74823131438024859, -18.25176868561973720 ) ) ;
#2817=CARTESIAN_POINT ( 'NONE',  ( 8.892440619315905792, 67.93243197801977828, 21.40021590834476228 ) ) ;
#2822=DIRECTION ( 'NONE',  ( -0.000000000000000000, -0.000000000000000000, 1.000000000000000000 ) ) ;
#2825=CARTESIAN_POINT ( 'NONE',  ( -71.68677369079009054, 77.11938847399009944, 12.77062708069394503 ) ) ;
#2831=FACE_OUTER_BOUND ( 'NONE', #3262, .T. ) ;
#2836=EDGE_LOOP ( 'NONE', ( #1934, #11109, #259, #8702, #10783, #6526 ) ) ;
#2838=CARTESIAN_POINT ( 'NONE',  ( -73.15625000204838102, 80.81189881250000440, -1.580522963032174394E-15 ) ) ;
#2839=EDGE_CURVE ( 'NONE', #11, #10526, #2084, .T. ) ;
#2841=DIRECTION ( 'NONE',  ( 1.000000000000000000, 0.000000000000000000, 0.000000000000000000 ) ) ;
#2866=EDGE_CURVE ( 'NONE', #3830, #1747, #8859, .T. ) ;
#2875=CARTESIAN_POINT ( 'NONE',  ( -13.03788829157083207, 70.42024943993379793, -19.68589793852361680 ) ) ;
#2877=ORIENTED_EDGE ( 'NONE', *, *, #5500, .F. ) ;
#2878=CARTESIAN_POINT ( 'NONE',  ( -78.87500000204838102, 80.81189881250001861, 10.69163855873948599 ) ) ;
#2879=ORIENTED_EDGE ( 'NONE', *, *, #2326, .T. ) ;
#2880=CARTESIAN_POINT ( 'NONE',  ( 20.91744440401235039, 76.33569358685066675, -13.03537739608741575 ) ) ;
#2882=ADVANCED_FACE ( 'NONE', ( #464 ), #6173, .F. ) ;
#2888=ORIENTED_EDGE ( 'NONE', *, *, #8211, .T. ) ;
#2896=CARTESIAN_POINT ( 'NONE',  ( -21.71522205163101660, 77.00056613986325260, 0.3292152594720888503 ) ) ;
#2900=DIRECTION ( 'NONE',  ( 1.000000000000000000, -0.000000000000000000, 0.000000000000000000 ) ) ;
#2904=CARTESIAN_POINT ( 'NONE',  ( -76.53125000204839523, 36.74823131438024859, -18.25176868561973720 ) ) ;
#2905=VECTOR ( 'NONE', #8919, 1000.000000000000000 ) ;
#2907=DIRECTION ( 'NONE',  ( -1.000000000000000000, -0.000000000000000000, -0.000000000000000000 ) ) ;
#2910=B_SPLINE_CURVE_WITH_KNOTS ( 'NONE', 1,
 ( #9446, #4001 ),
 .UNSPECIFIED., .F., .F.,
 ( 2, 2 ),
 ( 0.000000000000000000, 1.000000000000000000 ),
 .UNSPECIFIED. ) ;
#2913=CARTESIAN_POINT ( 'NONE',  ( -73.15625000204839523, 73.25176868561975141, -18.25176868561974430 ) ) ;
#2921=LINE ( 'NONE', #5124, #6731 ) ;
#2935=CARTESIAN_POINT ( 'NONE',  ( -16.15483550849972261, 72.60971644880963538, -17.79106955704961024 ) ) ;
#2939=EDGE_CURVE ( 'NONE', #9073, #10129, #1597, .T. ) ;
#2941=CARTESIAN_POINT ( 'NONE',  ( -75.87500000409677625, 55.00000000000000000, -24.99999999999999645 ) ) ;
#2942=ORIENTED_EDGE ( 'NONE', *, *, #11763, .T. ) ;
#2944=LINE ( 'NONE', #5644, #2121 ) ;
#2949=ORIENTED_EDGE ( 'NONE', *, *, #9448, .T. ) ;
#2956=CARTESIAN_POINT ( 'NONE',  ( -10.66763792956113832, 68.68038312560416614, 17.25573023236997372 ) ) ;
#2958=ORIENTED_EDGE ( 'NONE', *, *, #4675, .T. ) ;
#2961=EDGE_LOOP ( 'NONE', ( #2064, #2433, #6422, #10980 ) ) ;
#2963=CARTESIAN_POINT ( 'NONE',  ( -77.65625000204839523, 73.25176868561975141, -18.25176868561974430 ) ) ;
#2967=ORIENTED_EDGE ( 'NONE', *, *, #8112, .F. ) ;
#2972=EDGE_LOOP ( 'NONE', ( #11157, #1177, #234, #3771 ) ) ;
#2975=CARTESIAN_POINT ( 'NONE',  ( -73.43750000409677625, 37.32233047033631124, 17.67766952966369232 ) ) ;
#2978=DIRECTION ( 'NONE',  ( 1.000000000000000000, 0.000000000000000000, 0.000000000000000000 ) ) ;
#2979=ORIENTED_EDGE ( 'NONE', *, *, #2326, .F. ) ;
#2983=CARTESIAN_POINT ( 'NONE',  ( -78.50000000000000000, 55.00000000000000000, -24.99999999999999645 ) ) ;
#2984=DIRECTION ( 'NONE',  ( -0.000000000000000000, 1.000000000000000000, 0.000000000000000000 ) ) ;
#2985=VECTOR ( 'NONE', #10623, 1000.000000000000000 ) ;
#2986=CARTESIAN_POINT ( 'NONE',  ( -74.93750000409677625, 37.32233047033631124, 17.67766952966369232 ) ) ;
#2993=CARTESIAN_POINT ( 'NONE',  ( -72.50000000204839523, 29.18810118750000981, 10.69163855873950020 ) ) ;
#2997=CARTESIAN_POINT ( 'NONE',  ( -72.59375000204838102, 55.00000000000000000, 25.81189881249999729 ) ) ;
#2999=CARTESIAN_POINT ( 'NONE',  ( 6.621374545548222024, 66.85921098149330533, -22.01171010686805118 ) ) ;
#3003=CARTESIAN_POINT ( 'NONE',  ( 0.000000000000000000, 110.0000000000000000, 0.000000000000000000 ) ) ;
#3007=CARTESIAN_POINT ( 'NONE',  ( -74.18750000000007105, 37.32233047033641071, -17.67766952966358573 ) ) ;
#3012=CARTESIAN_POINT ( 'NONE',  ( -1.460760789256572600, 65.05635129456224774, 19.56749383220758887 ) ) ;
#3015=( GEOMETRIC_REPRESENTATION_CONTEXT ( 3 ) GLOBAL_UNCERTAINTY_ASSIGNED_CONTEXT ( ( #11693 ) ) GLOBAL_UNIT_ASSIGNED_CONTEXT ( ( #10298, #4737, #9225 ) ) REPRESENTATION_CONTEXT ( 'NONE', 'WORKASPACE' ) );
#3019=EDGE_CURVE ( 'NONE', #6717, #5255, #2317, .T. ) ;
#3022=CARTESIAN_POINT ( 'NONE',  ( -71.84375000204838102, 55.00000000000000000, -25.81189881249999729 ) ) ;
#3025=CARTESIAN_POINT ( 'NONE',  ( -79.81250000000004263, 72.67766952966367455, -17.67766952966367100 ) ) ;
#3029=CARTESIAN_POINT ( 'NONE',  ( -73.62500000204840944, 29.18810118750000626, -10.69163855873949132 ) ) ;
#3030=DIRECTION ( 'NONE',  ( 0.000000000000000000, 0.000000000000000000, -1.000000000000000000 ) ) ;
#3045=DIRECTION ( 'NONE',  ( 0.000000000000000000, 0.000000000000000000, 1.000000000000000000 ) ) ;
#3053=CARTESIAN_POINT ( 'NONE',  ( -25.03835002304701973, 79.78434740670915915, 3.387367328291911672 ) ) ;
#3056=CARTESIAN_POINT ( 'NONE',  ( -72.03125000204839523, 36.74823131438024859, -18.25176868561973720 ) ) ;
#3059=FACE_OUTER_BOUND ( 'NONE', #11831, .T. ) ;
#3068=CARTESIAN_POINT ( 'NONE',  ( -75.50000000000000000, 55.00000000000000000, -24.99999999999999645 ) ) ;
#3075=CARTESIAN_POINT ( 'NONE',  ( -15.87820011566687484, 72.30454950739435560, 13.62882577052523558 ) ) ;
#3078=CARTESIAN_POINT ( 'NONE',  ( -71.38989868722833876, 76.65063840437913711, 12.49999426730988361 ) ) ;
#3079=CARTESIAN_POINT ( 'NONE',  ( -77.65625000204838102, 80.81189881250000440, -1.580522963032174394E-15 ) ) ;
#3082=CARTESIAN_POINT ( 'NONE',  ( -72.31250000204839523, 29.18810118750000981, 10.69163855873950020 ) ) ;
#3084=EDGE_CURVE ( 'NONE', #5117, #8038, #2910, .T. ) ;
#3090=DIRECTION ( 'NONE',  ( 0.000000000000000000, 1.000000000000000000, 0.000000000000000000 ) ) ;
#3092=CARTESIAN_POINT ( 'NONE',  ( -72.50000000204836681, 44.30836144126052289, 25.81189881250000795 ) ) ;
#3105=ORIENTED_EDGE ( 'NONE', *, *, #6552, .F. ) ;
#3107=CARTESIAN_POINT ( 'NONE',  ( 39.99999999999999289, 55.00000000000000000, 24.99999999999999645 ) ) ;
#3111=ORIENTED_EDGE ( 'NONE', *, *, #6989, .F. ) ;
#3115=CARTESIAN_POINT ( 'NONE',  ( -79.15625000204839523, 73.25176868561975141, -18.25176868561974430 ) ) ;
#3116=FACE_BOUND ( 'NONE', #7219, .T. ) ;
#3119=CARTESIAN_POINT ( 'NONE',  ( -77.00000000409677625, 80.00000000000000000, -1.530808498934191324E-15 ) ) ;
#3121=CARTESIAN_POINT ( 'NONE',  ( 24.87203822307476031, 79.64205355216036253, 4.236592033986310568 ) ) ;
#3125=CARTESIAN_POINT ( 'NONE',  ( -73.34375000000007105, 65.35533905932732068, 24.99999999999986500 ) ) ;
#3127=CARTESIAN_POINT ( 'NONE',  ( -76.34375000000001421, 65.35533905932737753, 24.99999999999999645 ) ) ;
#3129=FACE_OUTER_BOUND ( 'NONE', #8174, .T. ) ;
#3133=CARTESIAN_POINT ( 'NONE',  ( -9.505256967967094184, 67.97321577359559797, 17.78506628848226256 ) ) ;
#3137=CARTESIAN_POINT ( 'NONE',  ( -75.78125000204838102, 55.00000000000000000, 25.81189881249999729 ) ) ;
#3147=FACE_OUTER_BOUND ( 'NONE', #6044, .T. ) ;
#3156=ORIENTED_EDGE ( 'NONE', *, *, #3084, .T. ) ;
#3162=PLANE ( 'NONE',  #10650 ) ;
#3169=EDGE_CURVE ( 'NONE', #11498, #10642, #3509, .T. ) ;
#3170=CARTESIAN_POINT ( 'NONE',  ( -74.65625000204839523, 73.25176868561975141, -18.25176868561974430 ) ) ;
#3171=CARTESIAN_POINT ( 'NONE',  ( -75.96875000000005684, 30.00000000000011013, 10.35533905932735088 ) ) ;
#3174=CARTESIAN_POINT ( 'NONE',  ( -78.78125000409679046, 65.35533905932737753, -24.99999999999999645 ) ) ;
#3175=LINE ( 'NONE', #11082, #11641 ) ;
#3183=CARTESIAN_POINT ( 'NONE',  ( -75.87500000000000000, 30.00000000000000355, 4.592425496802573578E-15 ) ) ;
#3189=CARTESIAN_POINT ( 'NONE',  ( 0.000000000000000000, 50.00000000000000000, 0.000000000000000000 ) ) ;
#3190=( NAMED_UNIT ( * ) SI_UNIT ( $, .STERADIAN. ) SOLID_ANGLE_UNIT ( ) );
#3192=CARTESIAN_POINT ( 'NONE',  ( 9.475534631369814775, 67.98327214991455492, -17.76592228101513271 ) ) ;
#3194=CARTESIAN_POINT ( 'NONE',  ( -79.15625000204838102, 80.81189881250000440, -1.580522963032174394E-15 ) ) ;
#3199=CARTESIAN_POINT ( 'NONE',  ( -79.62500000000001421, 79.99999999999997158, -1.530808498934189944E-15 ) ) ;
#3219=DIRECTION ( 'NONE',  ( -1.000000000000000000, -0.000000000000000000, -0.000000000000000000 ) ) ;
#3226=CARTESIAN_POINT ( 'NONE',  ( -74.56250000204839523, 80.81189881250000440, -10.69163855873948954 ) ) ;
#3227=CARTESIAN_POINT ( 'NONE',  ( -5.843944843092907071, 66.54774434410467165, 22.17515753471153772 ) ) ;
#3235=VECTOR ( 'NONE', #859, 1000.000000000000000 ) ;
#3241=CARTESIAN_POINT ( 'NONE',  ( -75.31250000000000000, 72.67766952966368876, -17.67766952966368876 ) ) ;
#3251=ORIENTED_EDGE ( 'NONE', *, *, #4742, .F. ) ;
#3252=CARTESIAN_POINT ( 'NONE',  ( 2.920128277213786205, 65.29083636825203030, 19.44520279024829179 ) ) ;
#3255=CARTESIAN_POINT ( 'NONE',  ( -74.00000000204840944, 44.30836144126053000, 25.81189881250000795 ) ) ;
#3257=DIRECTION ( 'NONE',  ( -1.000000000000000000, -0.000000000000000000, -0.000000000000000000 ) ) ;
#3262=EDGE_LOOP ( 'NONE', ( #1813, #3251, #4411, #11101 ) ) ;
#3263=CARTESIAN_POINT ( 'NONE',  ( 39.99999999999999289, 55.00000000000000000, -24.99999999999999645 ) ) ;
#3285=EDGE_CURVE ( 'NONE', #11173, #9573, #8534, .T. ) ;
#3286=CARTESIAN_POINT ( 'NONE',  ( -78.59375000204839523, 55.00000000000000000, 25.81189881249999729 ) ) ;
#3290=CARTESIAN_POINT ( 'NONE',  ( -72.03125000409679046, 44.64466094067262958, 25.00000000000001066 ) ) ;
#3297=CARTESIAN_POINT ( 'NONE',  ( -73.43750000000008527, 72.67766952966360350, 17.67766952966359284 ) ) ;
#3302=CARTESIAN_POINT ( 'NONE',  ( -75.40625000000000000, 65.35533905932737753, -24.99999999999999645 ) ) ;
#3303=CARTESIAN_POINT ( 'NONE',  ( 36.99999999999999289, 55.00000000000000000, 22.00000000000000000 ) ) ;
#3314=CARTESIAN_POINT ( 'NONE',  ( -78.12500000204839523, 44.30836144126049447, -25.81189881249999019 ) ) ;
#3315=ORIENTED_EDGE ( 'NONE', *, *, #5711, .T. ) ;
#3323=DIRECTION ( 'NONE',  ( 0.000000000000000000, 0.000000000000000000, 1.000000000000000000 ) ) ;
#3331=CARTESIAN_POINT ( 'NONE',  ( 39.99999999999999289, 39.99999999999999289, -19.99999999999999289 ) ) ;
#3333=DIRECTION ( 'NONE',  ( 0.000000000000000000, 0.000000000000000000, 1.000000000000000000 ) ) ;
#3339=DIRECTION ( 'NONE',  ( 0.000000000000000000, -0.000000000000000000, -1.000000000000000000 ) ) ;
#3343=CARTESIAN_POINT ( 'NONE',  ( -71.09375000409677625, 80.00000000000001421, -10.35533905932737753 ) ) ;
#3344=PLANE ( 'NONE',  #3624 ) ;
#3345=LINE ( 'NONE', #10761, #6555 ) ;
#3347=ORIENTED_EDGE ( 'NONE', *, *, #3649, .T. ) ;
#3350=DIRECTION ( 'NONE',  ( 1.000000000000000000, 0.000000000000000000, 0.000000000000000000 ) ) ;
#3355=CARTESIAN_POINT ( 'NONE',  ( -75.87500000204839523, 65.69163855873949842, 25.81189881250000440 ) ) ;
#3359=VERTEX_POINT ( 'NONE', #5908 ) ;
#3362=CARTESIAN_POINT ( 'NONE',  ( 39.99999999999999289, 55.00000000000000000, 0.000000000000000000 ) ) ;
#3363=DIRECTION ( 'NONE',  ( -0.000000000000000000, -0.000000000000000000, -1.000000000000000000 ) ) ;
#3365=CARTESIAN_POINT ( 'NONE',  ( 15.37375454209301395, 71.93308920591223909, -14.05578583284283312 ) ) ;
#3367=EDGE_LOOP ( 'NONE', ( #5483, #7810, #2551, #3347 ) ) ;
#3368=MECHANICAL_DESIGN_GEOMETRIC_PRESENTATION_REPRESENTATION('',(#8538),#11007);
#3372=CARTESIAN_POINT ( 'NONE',  ( -72.87500000409677625, 55.00000000000000000, -24.99999999999999645 ) ) ;
#3376=ORIENTED_EDGE ( 'NONE', *, *, #8735, .T. ) ;
#3383=CARTESIAN_POINT ( 'NONE',  ( -77.28125000204838102, 55.00000000000000000, 25.81189881249999729 ) ) ;
#3404=CARTESIAN_POINT ( 'NONE',  ( -70.87427368927673399, 76.65063840437987608, 12.49999426731031527 ) ) ;
#3405=FACE_OUTER_BOUND ( 'NONE', #249, .T. ) ;
#3415=CARTESIAN_POINT ( 'NONE',  ( -77.37500000204838102, 65.69163855873949842, 25.81189881250000440 ) ) ;
#3418=EDGE_CURVE ( 'NONE', #5411, #6717, #4247, .T. ) ;
#3425=CARTESIAN_POINT ( 'NONE',  ( 13.91855488460707058, 70.86244548763734485, -15.28271326984324929 ) ) ;
#3443=ORIENTED_EDGE ( 'NONE', *, *, #4044, .T. ) ;
#3446=CARTESIAN_POINT ( 'NONE',  ( -76.43750000204838102, 65.69163855873948421, -25.81189881250000440 ) ) ;
#3454=SURFACE_STYLE_FILL_AREA ( #6282 ) ;
#3472=CARTESIAN_POINT ( 'NONE',  ( -74.56250000409677625, 37.32233047033631124, -17.67766952966368166 ) ) ;
#3477=ORIENTED_EDGE ( 'NONE', *, *, #726, .T. ) ;
#3483=CARTESIAN_POINT ( 'NONE',  ( -78.59375000204839523, 36.74823131438026280, 18.25176868561974786 ) ) ;
#3488=CARTESIAN_POINT ( 'NONE',  ( 3.412284745132829311, 65.80390522347528304, 22.54555962154040927 ) ) ;
#3491=DIRECTION ( 'NONE',  ( -0.000000000000000000, -0.000000000000000000, 1.000000000000000000 ) ) ;
#3492=CARTESIAN_POINT ( 'NONE',  ( -77.75000000000000000, 55.00000000000000000, 24.99999999999999645 ) ) ;
#3493=CARTESIAN_POINT ( 'NONE',  ( -71.65625000204838102, 80.81189881250000440, -1.580522963032174394E-15 ) ) ;
#3506=CARTESIAN_POINT ( 'NONE',  ( -75.50000000204840944, 29.18810118750000981, 10.69163855873950020 ) ) ;
#3509=LINE ( 'NONE', #3331, #2985 ) ;
#3514=VERTEX_POINT ( 'NONE', #5910 ) ;
#3520=EDGE_CURVE ( 'NONE', #2575, #9843, #6872, .T. ) ;
#3526=EDGE_LOOP ( 'NONE', ( #9424, #10546, #698, #1425, #5062, #11118, #312, #648 ) ) ;
#3528=EDGE_CURVE ( 'NONE', #1709, #4282, #6633, .T. ) ;
#3534=CARTESIAN_POINT ( 'NONE',  ( -75.21875000204839523, 36.74823131438024859, -18.25176868561973720 ) ) ;
#3537=FACE_OUTER_BOUND ( 'NONE', #2019, .T. ) ;
#3543=LINE ( 'NONE', #1681, #885 ) ;
#3545=AXIS2_PLACEMENT_3D ( 'NONE', #2311, #9622, #9115 ) ;
#3547=CARTESIAN_POINT ( 'NONE',  ( -73.71875000204839523, 36.74823131438024859, -18.25176868561973720 ) ) ;
#3549=FACE_OUTER_BOUND ( 'NONE', #2260, .T. ) ;
#3556=CARTESIAN_POINT ( 'NONE',  ( -11.21107213742082109, 69.03605984126116368, -16.94742667234782374 ) ) ;
#3563=CARTESIAN_POINT ( 'NONE',  ( -74.65625000204838102, 80.81189881250000440, -1.580522963032174394E-15 ) ) ;
#3584=DIRECTION ( 'NONE',  ( -0.000000000000000000, -0.000000000000000000, -1.000000000000000000 ) ) ;
#3593=CARTESIAN_POINT ( 'NONE',  ( 39.99999999999999289, 55.00000000000000000, 5.249999999999998224 ) ) ;
#3596=CARTESIAN_POINT ( 'NONE',  ( -75.31250000204839523, 29.18810118750000626, -10.69163855873949309 ) ) ;
#3600=CARTESIAN_POINT ( 'NONE',  ( -77.37500000204838102, 80.81189881250001861, 10.69163855873948599 ) ) ;
#3602=CARTESIAN_POINT ( 'NONE',  ( 20.93592707265620945, 76.34962308819727639, 13.02666796807690552 ) ) ;
#3605=CARTESIAN_POINT ( 'NONE',  ( -76.81250000409679046, 72.67766952966368876, 17.67766952966368521 ) ) ;
#3615=CARTESIAN_POINT ( 'NONE',  ( -21.37442402976132882, 76.71451586203353656, 3.603759168105849398 ) ) ;
#3622=CARTESIAN_POINT ( 'NONE',  ( -77.18750000204839523, 65.69163855873949842, 25.81189881250000440 ) ) ;
#3624=AXIS2_PLACEMENT_3D ( 'NONE', #6236, #757, #816 ) ;
#3647=VECTOR ( 'NONE', #10191, 1000.000000000000000 ) ;
#3648=CARTESIAN_POINT ( 'NONE',  ( -74.56250000409677625, 37.32233047033631124, -17.67766952966368166 ) ) ;
#3649=EDGE_CURVE ( 'NONE', #30, #9521, #11261, .T. ) ;
#3650=EDGE_LOOP ( 'NONE', ( #10736, #9393 ) ) ;
#3651=CARTESIAN_POINT ( 'NONE',  ( 2.449293598294706513E-15, 50.00000000000000000, -20.00000000000000000 ) ) ;
#3655=CARTESIAN_POINT ( 'NONE',  ( -73.71875000204839523, 36.74823131438024859, -18.25176868561973720 ) ) ;
#3658=CARTESIAN_POINT ( 'NONE',  ( -74.46875000204839523, 80.81189881250000440, -1.580522963032174394E-15 ) ) ;
#3660=AXIS2_PLACEMENT_3D ( 'NONE', #296, #6611, #1317 ) ;
#3662=CARTESIAN_POINT ( 'NONE',  ( 2.148233841220928753, 65.58248926441827109, 22.64989133859231885 ) ) ;
#3665=CARTESIAN_POINT ( 'NONE',  ( -79.06250000000002842, 37.32233047033633966, 17.67766952966367100 ) ) ;
#3669=DIRECTION ( 'NONE',  ( 2.126576849575776229E-17, 0.9848077530122080203, -0.1736481776669307198 ) ) ;
#3676=CARTESIAN_POINT ( 'NONE',  ( -20.71225445595675296, 76.16273347894681933, 6.021655603152394676 ) ) ;
#3683=CARTESIAN_POINT ( 'NONE',  ( -72.59375000204838102, 36.74823131438026280, 18.25176868561974786 ) ) ;
#3684=ORIENTED_EDGE ( 'NONE', *, *, #1024, .F. ) ;
#3691=ORIENTED_EDGE ( 'NONE', *, *, #11404, .F. ) ;
#3699=CARTESIAN_POINT ( 'NONE',  ( 39.99999999999999289, 55.00000000000000000, -24.99999999999999645 ) ) ;
#3704=EDGE_LOOP ( 'NONE', ( #4229, #10467 ) ) ;
#3707=DIRECTION ( 'NONE',  ( 1.000000000000000000, 0.000000000000000000, 0.000000000000000000 ) ) ;
#3709=CARTESIAN_POINT ( 'NONE',  ( -71.93750000204838102, 65.69163855873948421, -25.81189881250000440 ) ) ;
#3712=CARTESIAN_POINT ( 'NONE',  ( -75.68750000204839523, 65.69163855873949842, 25.81189881250000440 ) ) ;
#3720=CARTESIAN_POINT ( 'NONE',  ( 14.99999999999999645, 5.000000000000000000, 20.00000000000000000 ) ) ;
#3722=CARTESIAN_POINT ( 'NONE',  ( -79.06250000000001421, 37.32233047033631124, 17.67766952966369232 ) ) ;
#3727=CARTESIAN_POINT ( 'NONE',  ( -18.57601780462385577, 74.41890655751923589, 10.34450647405109081 ) ) ;
#3735=CARTESIAN_POINT ( 'NONE',  ( -73.81250000204839523, 29.18810118750000626, -10.69163855873949309 ) ) ;
#3745=AXIS2_PLACEMENT_3D ( 'NONE', #2552, #9853, #5139 ) ;
#3746=ORIENTED_EDGE ( 'NONE', *, *, #6842, .T. ) ;
#3753=CYLINDRICAL_SURFACE ( 'NONE', #9172, 24.99999999999999645 ) ;
#3754=CARTESIAN_POINT ( 'NONE',  ( -72.50000000000000000, 55.00000000000000000, -24.99999999999999645 ) ) ;
#3755=EDGE_LOOP ( 'NONE', ( #7658, #7752, #4094, #4499, #2958, #6333, #5816, #5791, #8161, #11760, #11701, #8806, #3684, #11318 ) ) ;
#3760=PRODUCT ( 'Cast Iron Barrel & Hopper Casing', 'Cast Iron Barrel & Hopper Casing', '', ( #9119 ) ) ;
#3769=CARTESIAN_POINT ( 'NONE',  ( 2.782474192756827142E-15, 65.42943686846950868, -22.72062601704910634 ) ) ;
#3771=ORIENTED_EDGE ( 'NONE', *, *, #6458, .T. ) ;
#3773=CARTESIAN_POINT ( 'NONE',  ( -77.00000000204838102, 44.30836144126053000, 25.81189881250000795 ) ) ;
#3775=CARTESIAN_POINT ( 'NONE',  ( 25.22669093968800880, 79.94582849343181863, -1.700159177187467563 ) ) ;
#3780=DIRECTION ( 'NONE',  ( 0.000000000000000000, 0.000000000000000000, 1.000000000000000000 ) ) ;
#3783=CARTESIAN_POINT ( 'NONE',  ( -78.21875000000001421, 80.00000000000001421, -10.35533905932737753 ) ) ;
#3790=CARTESIAN_POINT ( 'NONE',  ( -19.43088458554904108, 75.10954819156191320, -8.928210389664046787 ) ) ;
#3798=CARTESIAN_POINT ( 'NONE',  ( -73.90625000204838102, 29.18810118750000271, 4.741568889096522788E-15 ) ) ;
#3803=ORIENTED_EDGE ( 'NONE', *, *, #3019, .F. ) ;
#3804=CARTESIAN_POINT ( 'NONE',  ( -73.25000000204839523, 65.69163855873948421, -25.81189881250000084 ) ) ;
#3809=ORIENTED_EDGE ( 'NONE', *, *, #485, .T. ) ;
#3813=VECTOR ( 'NONE', #2769, 1000.000000000000000 ) ;
#3817=CARTESIAN_POINT ( 'NONE',  ( -72.40625000000007105, 65.35533905932732068, -24.99999999999987921 ) ) ;
#3822=ADVANCED_FACE ( 'NONE', ( #2831 ), #7339, .F. ) ;
#3825=CARTESIAN_POINT ( 'NONE',  ( -77.46875000000005684, 30.00000000000010303, 10.35533905932735443 ) ) ;
#3827=EDGE_CURVE ( 'NONE', #2054, #10529, #4227, .T. ) ;
#3830=VERTEX_POINT ( 'NONE', #11380 ) ;
#3833=CARTESIAN_POINT ( 'NONE',  ( 0.000000000000000000, 110.0000000000000000, 0.000000000000000000 ) ) ;
#3834=DIRECTION ( 'NONE',  ( 0.000000000000000000, 1.000000000000000000, 0.000000000000000000 ) ) ;
#3836=CARTESIAN_POINT ( 'NONE',  ( -73.43750000204839523, 65.69163855873948421, -25.81189881250000440 ) ) ;
#3838=ORIENTED_EDGE ( 'NONE', *, *, #6586, .F. ) ;
#3839=CARTESIAN_POINT ( 'NONE',  ( -75.87500000204839523, 80.81189881250001861, 10.69163855873948599 ) ) ;
#3840=EDGE_LOOP ( 'NONE', ( #3803, #4533, #10596 ) ) ;
#3843=DIRECTION ( 'NONE',  ( -1.000000000000000000, -0.000000000000000000, -0.000000000000000000 ) ) ;
#3854=CARTESIAN_POINT ( 'NONE',  ( -5.682122240792035761, 66.13352472168112683, 18.97764918900208997 ) ) ;
#3865=CARTESIAN_POINT ( 'NONE',  ( -73.06250000204840944, 80.81189881250001861, 10.69163855873948599 ) ) ;
#3873=DIRECTION ( 'NONE',  ( 0.000000000000000000, 0.000000000000000000, 1.000000000000000000 ) ) ;
#3880=CARTESIAN_POINT ( 'NONE',  ( -72.21875000000008527, 79.99999999999988631, -10.35533905932732601 ) ) ;
#3890=CARTESIAN_POINT ( 'NONE',  ( 0.000000000000000000, 50.52094453300079380, 0.000000000000000000 ) ) ;
#3894=CARTESIAN_POINT ( 'NONE',  ( -5.866463102745652414, 66.55608005278446626, -22.17084374085253629 ) ) ;
#3897=CARTESIAN_POINT ( 'NONE',  ( -72.40625000204839523, 36.74823131438026280, 18.25176868561974786 ) ) ;
#3899=CARTESIAN_POINT ( 'NONE',  ( 21.59285841830472918, 76.88861624364108138, -12.08424295940928772 ) ) ;
#3906=CARTESIAN_POINT ( 'NONE',  ( -79.62500000000000000, 80.00000000000000000, -1.530808498934191324E-15 ) ) ;
#3914=DIRECTION ( 'NONE',  ( 0.000000000000000000, 0.000000000000000000, -1.000000000000000000 ) ) ;
#3917=EDGE_CURVE ( 'NONE', #3830, #10858, #630, .T. ) ;
#3919=CARTESIAN_POINT ( 'NONE',  ( -75.59375000204839523, 55.00000000000000000, 25.81189881249999729 ) ) ;
#3925=CARTESIAN_POINT ( 'NONE',  ( -72.21875000409676204, 65.35533905932712173, 25.00000000000025580 ) ) ;
#3927=DIRECTION ( 'NONE',  ( 0.000000000000000000, 1.000000000000000000, 0.000000000000000000 ) ) ;
#3933=CARTESIAN_POINT ( 'NONE',  ( -76.25000000409677625, 30.00000000000000355, 4.592425496802573578E-15 ) ) ;
#3942=CARTESIAN_POINT ( 'NONE',  ( -75.12500000409677625, 55.00000000000000000, 24.99999999999999645 ) ) ;
#3947=CARTESIAN_POINT ( 'NONE',  ( 36.99999999999999289, 55.00000000000000000, -22.00000000000000000 ) ) ;
#3951=CARTESIAN_POINT ( 'NONE',  ( -24.49417083054724742, 79.31944638913208223, 5.853031391697339991 ) ) ;
#3955=CARTESIAN_POINT ( 'NONE',  ( -72.78125000204839523, 73.25176868561975141, 18.25176868561974075 ) ) ;
#3957=CARTESIAN_POINT ( 'NONE',  ( 25.18797318253816186, 79.91260864020590304, -2.131801228107524704 ) ) ;
#3960=EDGE_CURVE ( 'NONE', #4962, #4282, #10427, .T. ) ;
#3963=CARTESIAN_POINT ( 'NONE',  ( -75.50000000000001421, 54.99999999999944578, -24.99999999999999645 ) ) ;
#3966=ADVANCED_FACE ( 'NONE', ( #4997 ), #2314, .T. ) ;
#3967=CARTESIAN_POINT ( 'NONE',  ( -77.75000000000000000, 55.00000000000000000, 24.99999999999999645 ) ) ;
#3971=ORIENTED_EDGE ( 'NONE', *, *, #11621, .F. ) ;
#3973=CARTESIAN_POINT ( 'NONE',  ( -72.68750000000007105, 37.32233047033641071, -17.67766952966357863 ) ) ;
#3979=CARTESIAN_POINT ( 'NONE',  ( -79.25000000204839523, 80.81189881250000440, -10.69163855873948954 ) ) ;
#3980=ORIENTED_EDGE ( 'NONE', *, *, #2392, .T. ) ;
#3982=CARTESIAN_POINT ( 'NONE',  ( -74.75000000204840944, 65.69163855873948421, -25.81189881250000440 ) ) ;
#3983=CARTESIAN_POINT ( 'NONE',  ( 39.99999999999999289, 55.00000000000000000, 0.000000000000000000 ) ) ;
#3986=CARTESIAN_POINT ( 'NONE',  ( -77.56250000409679046, 37.32233047033631124, -17.67766952966368166 ) ) ;
#3987=VERTEX_POINT ( 'NONE', #9771 ) ;
#3988=CARTESIAN_POINT ( 'NONE',  ( 14.99999999999999645, 39.99999999999999289, -20.00000000000000000 ) ) ;
#4001=CARTESIAN_POINT ( 'NONE',  ( -78.87500000409677625, 55.00000000000000000, -24.99999999999999645 ) ) ;
#4009=DIRECTION ( 'NONE',  ( 0.000000000000000000, 0.000000000000000000, -1.000000000000000000 ) ) ;
#4016=CARTESIAN_POINT ( 'NONE',  ( -77.37500000409677625, 55.00000000000000000, -24.99999999999999645 ) ) ;
#4024=EDGE_CURVE ( 'NONE', #9967, #2595, #2657, .T. ) ;
#4027=CARTESIAN_POINT ( 'NONE',  ( -77.84375000000001421, 65.35533905932737753, 24.99999999999999645 ) ) ;
#4030=ORIENTED_EDGE ( 'NONE', *, *, #8000, .T. ) ;
#4037=DIRECTION ( 'NONE',  ( 1.000000000000000000, 0.000000000000000000, 0.000000000000000000 ) ) ;
#4040=VERTEX_POINT ( 'NONE', #8043 ) ;
#4043=CARTESIAN_POINT ( 'NONE',  ( -73.25000000204839523, 65.69163855873948421, -25.81189881250000440 ) ) ;
#4044=EDGE_CURVE ( 'NONE', #7325, #1879, #6924, .T. ) ;
#4049=CARTESIAN_POINT ( 'NONE',  ( -77.75000000409677625, 30.00000000000000355, 4.592425496802573578E-15 ) ) ;
#4057=AXIS2_PLACEMENT_3D ( 'NONE', #4487, #8138, #10819 ) ;
#4062=CARTESIAN_POINT ( 'NONE',  ( -76.15625000409677625, 30.00000000000000355, -10.35533905932738108 ) ) ;
#4073=CARTESIAN_POINT ( 'NONE',  ( -75.03125000204839523, 36.74823131438024859, -18.25176868561973720 ) ) ;
#4074=CARTESIAN_POINT ( 'NONE',  ( -25.19064713987262394, 79.91490204074258941, 2.105276644174951084 ) ) ;
#4077=CARTESIAN_POINT ( 'NONE',  ( -77.75000000409677625, 30.00000000000000355, 4.592425496802573578E-15 ) ) ;
#4083=CARTESIAN_POINT ( 'NONE',  ( -76.90625000000000000, 65.35533905932737753, -24.99999999999999645 ) ) ;
#4086=ORIENTED_EDGE ( 'NONE', *, *, #4187, .F. ) ;
#4092=CARTESIAN_POINT ( 'NONE',  ( 15.85754866970926358, 72.28899002677383123, 13.64810891474729004 ) ) ;
#4094=ORIENTED_EDGE ( 'NONE', *, *, #9085, .T. ) ;
#4097=CARTESIAN_POINT ( 'NONE',  ( -72.50000000204839523, 44.30836144126053000, 25.81189881250000795 ) ) ;
#4099=CARTESIAN_POINT ( 'NONE',  ( -79.71875000000000000, 79.99999999999998579, -10.35533905932736332 ) ) ;
#4123=CARTESIAN_POINT ( 'NONE',  ( -77.00000000204839523, 44.30836144126052289, 25.81189881250000795 ) ) ;
#4124=CARTESIAN_POINT ( 'NONE',  ( -25.23647670057383152, 79.95418391132277236, -1.735782755942627542 ) ) ;
#4127=CARTESIAN_POINT ( 'NONE',  ( -72.68750000409677625, 72.67766952966368876, -17.67766952966368876 ) ) ;
#4135=EDGE_LOOP ( 'NONE', ( #7150, #7256, #5213, #3691 ) ) ;
#4138=CARTESIAN_POINT ( 'NONE',  ( -73.34375000000001421, 65.35533905932737753, 24.99999999999999645 ) ) ;
#4146=ORIENTED_EDGE ( 'NONE', *, *, #10001, .F. ) ;
#4147=CARTESIAN_POINT ( 'NONE',  ( 6.021660879821575385, 66.27766067927709059, -18.89023547443478179 ) ) ;
#4152=CARTESIAN_POINT ( 'NONE',  ( -74.18750000204839523, 65.69163855873949842, 25.81189881250000440 ) ) ;
#4154=DIRECTION ( 'NONE',  ( 1.000000000000000000, 0.000000000000000000, 0.000000000000000000 ) ) ;
#4157=CIRCLE ( 'NONE', #10455, 5.000000000000000000 ) ;
#4180=ORIENTED_EDGE ( 'NONE', *, *, #8437, .T. ) ;
#4184=CARTESIAN_POINT ( 'NONE',  ( -78.31250000204839523, 29.18810118750000981, 10.69163855873950020 ) ) ;
#4185=CARTESIAN_POINT ( 'NONE',  ( -1.625240267017640655E-20, 65.42943686846950868, 22.72062601704910634 ) ) ;
#4187=EDGE_CURVE ( 'NONE', #4200, #896, #2706, .T. ) ;
#4188=ADVANCED_FACE ( 'NONE', ( #5584 ), #5349, .F. ) ;
#4190=CARTESIAN_POINT ( 'NONE',  ( -73.25000000409677625, 30.00000000000000355, 4.592425496802573578E-15 ) ) ;
#4200=VERTEX_POINT ( 'NONE', #9111 ) ;
#4202=CARTESIAN_POINT ( 'NONE',  ( -76.62500000000000000, 80.00000000000000000, -1.530808498934191324E-15 ) ) ;
#4212=CARTESIAN_POINT ( 'NONE',  ( 19.90507239772531634, 75.49690331019444045, 7.999200882884572650 ) ) ;
#4213=CARTESIAN_POINT ( 'NONE',  ( -78.96875000204839523, 73.25176868561975141, 18.25176868561974075 ) ) ;
#4218=CARTESIAN_POINT ( 'NONE',  ( -75.12500000409677625, 55.00000000000000000, 24.99999999999999645 ) ) ;
#4227=B_SPLINE_CURVE_WITH_KNOTS ( 'NONE', 3,
 ( #10127, #8170, #2776, #10010, #1087, #10912, #5472, #1928, #4575, #11018, #5601, #8284, #8115, #124, #3556, #1805, #1754, #7227, #10855, #6565, #9120, #2661, #904, #8230, #9239, #3790, #1026, #7458, #5532, #9181, #11084, #10194, #10066, #4689, #4515, #2896, #845, #2724, #5, #11811, #3615, #7283, #5656, #6435, #3676, #9292, #1866, #4633, #62, #3727, #7391, #8339, #2168, #2046, #3075, #8404, #8525, #5722, #7632, #2956, #3133, #187, #9602, #3854, #6621, #7748, #11140, #309, #11202, #3012, #9418, #8648 ),
 .UNSPECIFIED., .F., .F.,
 ( 4, 2, 2, 2, 2, 2, 2, 2, 2, 2, 2, 2, 2, 2, 2, 2, 2, 2, 2, 2, 2, 2, 2, 2, 2, 2, 2, 2, 2, 2, 2, 2, 2, 2, 2, 4 ),
 ( 0.06444559019126132327, 0.06662592794032556887, 0.06771609681485769860, 0.06880626568938981447, 0.07098660343845407394, 0.07316694118751831954, 0.07534727893658257902, 0.07752761668564682462, 0.08188829218377530195, 0.08406862993283956142, 0.08624896768190382090, 0.08842930543096806650, 0.08951947430550019624, 0.09060964318003232598, 0.09497031867816085882, 0.09606048755269300243, 0.09715065642722511829, 0.09933099417628937777, 0.1004211630508214936, 0.1015113319253536234, 0.1036916696744178829, 0.1047818385489500126, 0.1058720074234821285, 0.1080523451725464018, 0.1102326829216106613, 0.1113228517961427910, 0.1124130206706749346, 0.1167736961688034397, 0.1189540339178676853, 0.1211343716669319170, 0.1254950471650604360, 0.1276753849141247232, 0.1298557226631889550, 0.1309458915377210986, 0.1320360604122532422, 0.1342163981613174739 ),
 .UNSPECIFIED. ) ;
#4229=ORIENTED_EDGE ( 'NONE', *, *, #11821, .F. ) ;
#4232=CARTESIAN_POINT ( 'NONE',  ( -75.21875000204839523, 36.74823131438024859, -18.25176868561973720 ) ) ;
#4240=VECTOR ( 'NONE', #2345, 1000.000000000000000 ) ;
#4246=CARTESIAN_POINT ( 'NONE',  ( -77.28125000204839523, 73.25176868561975141, 18.25176868561974075 ) ) ;
#4247=( BOUNDED_CURVE ( )  B_SPLINE_CURVE ( 2, ( #7586, #11214, #3025, #4099, #3199, #10495, #6693, #2119, #5796 ),
 .UNSPECIFIED., .F., .T. ) 
 B_SPLINE_CURVE_WITH_KNOTS ( ( 3, 2, 2, 2, 3 ),
 ( 0.000000000000000000, 0.01979916996583446290, 0.03959833993166892580, 0.05939750989750339216, 0.07919667986333785159 ),
 .UNSPECIFIED. ) 
 CURVE ( )  GEOMETRIC_REPRESENTATION_ITEM ( )  RATIONAL_B_SPLINE_CURVE ( ( 1.000000000000000000, 0.9238795325112868495, 1.000000000000000000, 0.9238795325112868495, 1.000000000000000000, 0.9238795325112868495, 1.000000000000000000, 0.9238795325112868495, 1.000000000000000000 ) ) 
 REPRESENTATION_ITEM ( '' )  );
#4250=ORIENTED_EDGE ( 'NONE', *, *, #5500, .T. ) ;
#4251=CARTESIAN_POINT ( 'NONE',  ( -72.87500000409677625, 55.00000000000000000, -24.99999999999999645 ) ) ;
#4252=LINE ( 'NONE', #9926, #1705 ) ;
#4253=CARTESIAN_POINT ( 'NONE',  ( -71.46875000409677625, 44.64466094067286406, -25.00000000000024869 ) ) ;
#4261=LINE ( 'NONE', #7799, #4240 ) ;
#4262=CARTESIAN_POINT ( 'NONE',  ( -77.56250000204838102, 80.81189881250001861, 10.69163855873948599 ) ) ;
#4263=CARTESIAN_POINT ( 'NONE',  ( 0.000000000000000000, -30.00000000000000000, 0.000000000000000000 ) ) ;
#4271=FACE_OUTER_BOUND ( 'NONE', #8596, .T. ) ;
#4273=CARTESIAN_POINT ( 'NONE',  ( 17.18324390207781960, 73.31587886235929830, -12.20234056926149080 ) ) ;
#4277=DIRECTION ( 'NONE',  ( 0.000000000000000000, 0.000000000000000000, -1.000000000000000000 ) ) ;
#4282=VERTEX_POINT ( 'NONE', #7564 ) ;
#4284=EDGE_CURVE ( 'NONE', #2595, #10896, #919, .T. ) ;
#4289=CARTESIAN_POINT ( 'NONE',  ( -78.59375000204839523, 36.74823131438026280, 18.25176868561974786 ) ) ;
#4290=ORIENTED_EDGE ( 'NONE', *, *, #5660, .T. ) ;
#4304=ORIENTED_EDGE ( 'NONE', *, *, #8942, .T. ) ;
#4305=CARTESIAN_POINT ( 'NONE',  ( -73.81250000409677625, 72.67766952966368876, 17.67766952966368521 ) ) ;
#4318=DIRECTION ( 'NONE',  ( -1.000000000000000000, -0.000000000000000000, -0.000000000000000000 ) ) ;
#4319=CARTESIAN_POINT ( 'NONE',  ( -78.87500000204838102, 65.69163855873949842, 25.81189881250000440 ) ) ;
#4324=EDGE_CURVE ( 'NONE', #388, #6710, #2944, .T. ) ;
#4329=CARTESIAN_POINT ( 'NONE',  ( -77.09375000409677625, 80.00000000000001421, -10.35533905932737753 ) ) ;
#4333=ADVANCED_FACE ( 'NONE', ( #8577 ), #1975, .F. ) ;
#4334=CARTESIAN_POINT ( 'NONE',  ( 19.13801014043440318, 74.86951949782532267, -9.538400742199257820 ) ) ;
#4335=CARTESIAN_POINT ( 'NONE',  ( -71.59560441993424718, 80.81189881250001861, 6.916273537586018705 ) ) ;
#4347=CIRCLE ( 'NONE', #5119, 5.249999999999998224 ) ;
#4349=CARTESIAN_POINT ( 'NONE',  ( 0.000000000000000000, -24.99999999999999645, 0.000000000000000000 ) ) ;
#4354=CARTESIAN_POINT ( 'NONE',  ( -78.31250000204838102, 29.18810118750000626, -10.69163855873949309 ) ) ;
#4366=CARTESIAN_POINT ( 'NONE',  ( 39.99999999999999289, 55.00000000000000000, 24.99999999999999645 ) ) ;
#4371=CARTESIAN_POINT ( 'NONE',  ( -75.21875000409677625, 65.35533905932737753, 24.99999999999999645 ) ) ;
#4376=ORIENTED_EDGE ( 'NONE', *, *, #6831, .F. ) ;
#4382=CARTESIAN_POINT ( 'NONE',  ( -74.93750000204839523, 65.69163855873948421, -25.81189881250000440 ) ) ;
#4385=CARTESIAN_POINT ( 'NONE',  ( 14.99999999999999645, 55.00000000000000000, 0.000000000000000000 ) ) ;
#4387=CARTESIAN_POINT ( 'NONE',  ( 24.78347237616896237, 79.56634503030461758, 4.655107467241123231 ) ) ;
#4388=AXIS2_PLACEMENT_3D ( 'NONE', #8676, #7897, #7002 ) ;
#4390=CARTESIAN_POINT ( 'NONE',  ( -71.03052368859394505, 76.88501343918500197, 12.63531067400213104 ) ) ;
#4391=CARTESIAN_POINT ( 'NONE',  ( 36.99999999999999289, 55.00000000000000000, 5.249999999999998224 ) ) ;
#4394=CARTESIAN_POINT ( 'NONE',  ( 36.99999999999999289, 55.00000000000000000, 0.000000000000000000 ) ) ;
#4400=UNCERTAINTY_MEASURE_WITH_UNIT (LENGTH_MEASURE( 1.000000000000000082E-05 ), #4417, 'distance_accuracy_value', 'NONE');
#4411=ORIENTED_EDGE ( 'NONE', *, *, #5652, .F. ) ;
#4413=CARTESIAN_POINT ( 'NONE',  ( -76.71875000204839523, 36.74823131438024859, -18.25176868561973720 ) ) ;
#4417=( LENGTH_UNIT ( ) NAMED_UNIT ( * ) SI_UNIT ( .MILLI., .METRE. ) );
#4425=VECTOR ( 'NONE', #7363, 1000.000000000000000 ) ;
#4433=PLANE ( 'NONE',  #4057 ) ;
#4435=VECTOR ( 'NONE', #5668, 1000.000000000000000 ) ;
#4436=ORIENTED_EDGE ( 'NONE', *, *, #8942, .F. ) ;
#4442=DIRECTION ( 'NONE',  ( 2.126576849575776229E-17, 0.9848077530122080203, -0.1736481776669307198 ) ) ;
#4444=CARTESIAN_POINT ( 'NONE',  ( -77.00000000204838102, 29.18810118750000981, 10.69163855873950020 ) ) ;
#4455=DIRECTION ( 'NONE',  ( 1.000000000000000000, 0.000000000000000000, 0.000000000000000000 ) ) ;
#4460=EDGE_CURVE ( 'NONE', #10478, #9989, #7990, .T. ) ;
#4470=CARTESIAN_POINT ( 'NONE',  ( -74.84375000204839523, 73.25176868561975141, -18.25176868561974430 ) ) ;
#4471=ORIENTED_EDGE ( 'NONE', *, *, #10184, .T. ) ;
#4485=CARTESIAN_POINT ( 'NONE',  ( -76.34375000000005684, 65.35533905932732068, 24.99999999999990052 ) ) ;
#4487=CARTESIAN_POINT ( 'NONE',  ( 0.000000000000000000, 5.000000000000000000, 0.000000000000000000 ) ) ;
#4496=CARTESIAN_POINT ( 'NONE',  ( -78.68750000204838102, 44.30836144126053000, 25.81189881250000795 ) ) ;
#4499=ORIENTED_EDGE ( 'NONE', *, *, #10336, .T. ) ;
#4500=CARTESIAN_POINT ( 'NONE',  ( -75.12500000204838102, 29.18810118750000626, -10.69163855873949309 ) ) ;
#4502=CARTESIAN_POINT ( 'NONE',  ( 6.634799041927093910, 66.87503529737901431, 22.00033049848320488 ) ) ;
#4505=CARTESIAN_POINT ( 'NONE',  ( -77.00000000409677625, 80.00000000000000000, -1.530808498934191324E-15 ) ) ;
#4507=ORIENTED_EDGE ( 'NONE', *, *, #10614, .F. ) ;
#4515=CARTESIAN_POINT ( 'NONE',  ( -21.71309743435359962, 76.99877995635615946, -0.7660633642738442495 ) ) ;
#4523=CARTESIAN_POINT ( 'NONE',  ( -72.40625000204838102, 29.18810118750000271, 4.741568889096522788E-15 ) ) ;
#4533=ORIENTED_EDGE ( 'NONE', *, *, #3418, .F. ) ;
#4557=CARTESIAN_POINT ( 'NONE',  ( -71.75000000204838102, 80.81189881250001861, -10.69163855873949132 ) ) ;
#4561=CARTESIAN_POINT ( 'NONE',  ( -74.84375000204839523, 55.00000000000000000, -25.81189881249999729 ) ) ;
#4562=ORIENTED_EDGE ( 'NONE', *, *, #10075, .T. ) ;
#4563=CARTESIAN_POINT ( 'NONE',  ( 24.28641463743580786, 79.14216019722405804, 6.705329215194802295 ) ) ;
#4575=CARTESIAN_POINT ( 'NONE',  ( -5.679186637561253193, 66.13248820997100097, -18.97822730947832781 ) ) ;
#4581=CARTESIAN_POINT ( 'NONE',  ( -79.25000000204838102, 65.69163855873948421, -25.81189881250000440 ) ) ;
#4587=ORIENTED_EDGE ( 'NONE', *, *, #140, .F. ) ;
#4590=ORIENTED_EDGE ( 'NONE', *, *, #2362, .T. ) ;
#4597=EDGE_LOOP ( 'NONE', ( #4290, #7413, #1314, #4304 ) ) ;
#4598=CARTESIAN_POINT ( 'NONE',  ( -76.81250000000007105, 72.67766952966361771, -17.67766952966362126 ) ) ;
#4611=CARTESIAN_POINT ( 'NONE',  ( -72.31250000204839523, 29.18810118750000626, -10.69163855873949309 ) ) ;
#4614=CARTESIAN_POINT ( 'NONE',  ( -77.84375000204839523, 55.00000000000000000, -25.81189881249999729 ) ) ;
#4616=ORIENTED_EDGE ( 'NONE', *, *, #5340, .F. ) ;
#4625=ORIENTED_EDGE ( 'NONE', *, *, #7410, .F. ) ;
#4633=CARTESIAN_POINT ( 'NONE',  ( -19.45868386605759426, 75.13175751020747839, 8.896918319219480509 ) ) ;
#4641=CARTESIAN_POINT ( 'NONE',  ( -77.75000000204839523, 65.69163855873948421, -25.81189881250000440 ) ) ;
#4652=LINE ( 'NONE', #10033, #5085 ) ;
#4654=CARTESIAN_POINT ( 'NONE',  ( -15.00000000000000355, 5.000000000000000000, 30.00000000000000711 ) ) ;
#4656=LINE ( 'NONE', #3699, #4425 ) ;
#4665=CARTESIAN_POINT ( 'NONE',  ( -72.31250000204839523, 29.18810118750000626, -10.69163855873949132 ) ) ;
#4668=CARTESIAN_POINT ( 'NONE',  ( -72.78125000204838102, 55.00000000000000000, 25.81189881249999729 ) ) ;
#4671=CARTESIAN_POINT ( 'NONE',  ( -78.21875000204839523, 29.18810118750000271, 4.741568889096522788E-15 ) ) ;
#4673=CARTESIAN_POINT ( 'NONE',  ( 21.37139390916209436, 76.70668867414399017, -12.40776174393255005 ) ) ;
#4675=EDGE_CURVE ( 'NONE', #6797, #7233, #9207, .T. ) ;
#4681=CARTESIAN_POINT ( 'NONE',  ( -78.87500000000000000, 30.00000000000000355, 4.592425496802573578E-15 ) ) ;
#4687=EDGE_CURVE ( 'NONE', #847, #7502, #10401, .T. ) ;
#4689=CARTESIAN_POINT ( 'NONE',  ( -21.66859339435655230, 76.96133620317469592, -1.491344961900184174 ) ) ;
#4695=CARTESIAN_POINT ( 'NONE',  ( -73.71875000409679046, 65.35533905932720700, 25.00000000000016698 ) ) ;
#4698=( BOUNDED_SURFACE ( )  B_SPLINE_SURFACE ( 1, 2, ( 
 ( #7060, #9730, #5309, #681, #8901, #9793, #1586, #5194, #8847, #6335, #4289, #11522, #8964, #4354, #6996, #11706, #7947, #1530, #7173, #625, #10797, #11581, #738, #5254, #3383, #10619, #2668, #10680, #2430, #2493, #4413, #6158, #8005, #3446, #7118, #9908, #10743, #6216, #8064, #9848, #10860, #1640, #2608, #3506, #9964, #11757, #4232, #1704, #5368, #9020, #4470, #8122, #3563, #7892, #7235, #5136, #8784, #565, #10202, #1812, #3798, #3735, #10920, #2732, #6390, #1995, #13, #5480, #2838, #3865, #9075, #5665, #9187, #8413, #3683, #10018, #4523, #7401, #8178, #851, #9129, #9302, #910, #6506, #5608, #71, #2782 ),
 ( #1096, #4581, #5425, #9247, #7526, #4760, #6629, #196, #8237, #7346, #10971, #1936, #976, #5541, #6444, #10074, #1873, #4641, #2963, #8293, #11817, #1035, #11029, #3622, #8349, #10135, #4699, #7468, #134, #11092, #2904, #6573, #11148, #1760, #7290, #7814, #6689, #254, #4825, #9549, #3919, #6753, #7584, #2117, #1344, #10320, #377, #10434, #11387, #3982, #5974, #11445, #11211, #1156, #10381, #4152, #2177, #3255, #317, #5845, #9486, #8711, #8657, #7641, #1276, #4043, #5794, #11271, #5064, #9610, #8478, #436, #5008, #4097, #4945, #3082, #2298, #9426, #495, #6806, #3022, #8533, #6868, #1216, #10259, #7699, #8601 ) ),
 .UNSPECIFIED., .F., .F., .T. ) 
 B_SPLINE_SURFACE_WITH_KNOTS ( ( 2, 2 ),
 ( 3, 2, 2, 2, 2, 2, 2, 2, 2, 2, 2, 2, 2, 2, 2, 2, 2, 2, 2, 2, 2, 2, 2, 2, 2, 2, 2, 2, 2, 2, 2, 2, 2, 2, 2, 2, 2, 2, 2, 2, 2, 2, 2, 3 ),
 ( 0.000000000000000000, 1.000000000000000000 ),
 ( 0.000000000000000000, 0.02083333333333333218, 0.04166666666666666435, 0.06250000000000000000, 0.08333333333333332871, 0.1041666666666666713, 0.1250000000000000000, 0.1458333333333333426, 0.1666666666666666574, 0.1875000000000000000, 0.2083333333333333426, 0.2291666666666666574, 0.2500000000000000000, 0.2708333333333333148, 0.2916666666666666852, 0.3125000000000000000, 0.3333333333333333148, 0.3541666666666666852, 0.3750000000000000000, 0.3958333333333333148, 0.4166666666666666852, 0.4375000000000000000, 0.4583333333333333148, 0.4791666666666666852, 0.5000000000000000000, 0.5208333333333333703, 0.5416666666666666297, 0.5625000000000000000, 0.5833333333333333703, 0.6041666666666666297, 0.6250000000000000000, 0.6458333333333333703, 0.6666666666666666297, 0.6875000000000000000, 0.7083333333333333703, 0.7291666666666666297, 0.7500000000000000000, 0.7708333333333333703, 0.7916666666666666297, 0.8125000000000000000, 0.8333333333333333703, 0.8541666666666666297, 0.8750000000000000000, 0.8888490476107191451 ),
 .UNSPECIFIED. ) 
 GEOMETRIC_REPRESENTATION_ITEM ( )  RATIONAL_B_SPLINE_SURFACE ( (
 ( 1.000000000000000000, 0.9238795325112867385, 1.000000000000000000, 0.9238795325112867385, 1.000000000000000000, 0.9238795325112867385, 1.000000000000000000, 0.9238795325112867385, 1.000000000000000000, 0.9238795325112867385, 1.000000000000000000, 0.9238795325112867385, 1.000000000000000000, 0.9238795325112867385, 1.000000000000000000, 0.9238795325112867385, 1.000000000000000000, 0.9238795325112867385, 1.000000000000000000, 0.9238795325112867385, 1.000000000000000000, 0.9238795325112867385, 1.000000000000000000, 0.9238795325112867385, 1.000000000000000000, 0.9238795325112867385, 1.000000000000000000, 0.9238795325112867385, 1.000000000000000000, 0.9238795325112867385, 1.000000000000000000, 0.9238795325112867385, 1.000000000000000000, 0.9238795325112867385, 1.000000000000000000, 0.9238795325112867385, 1.000000000000000000, 0.9238795325112867385, 1.000000000000000000, 0.9238795325112867385, 1.000000000000000000, 0.9238795325112867385, 1.000000000000000000, 0.9238795325112867385, 1.000000000000000000, 0.9238795325112867385, 1.000000000000000000, 0.9238795325112867385, 1.000000000000000000, 0.9238795325112867385, 1.000000000000000000, 0.9238795325112867385, 1.000000000000000000, 0.9238795325112867385, 1.000000000000000000, 0.9238795325112867385, 1.000000000000000000, 0.9238795325112867385, 1.000000000000000000, 0.9238795325112867385, 1.000000000000000000, 0.9238795325112867385, 1.000000000000000000, 0.9238795325112867385, 1.000000000000000000, 0.9238795325112867385, 1.000000000000000000, 0.9238795325112867385, 1.000000000000000000, 0.9238795325112867385, 1.000000000000000000, 0.9238795325112867385, 1.000000000000000000, 0.9238795325112867385, 1.000000000000000000, 0.9238795325112867385, 1.000000000000000000, 0.9238795325112867385, 1.000000000000000000, 0.9238795325112867385, 1.000000000000000000, 0.9238795325112867385, 1.000000000000000000, 0.9238795325112867385, 1.000000000000000000, 0.9493985930367334625, 0.9660721903170175207),
 ( 1.000000000000000000, 0.9238795325112867385, 1.000000000000000000, 0.9238795325112867385, 1.000000000000000000, 0.9238795325112867385, 1.000000000000000000, 0.9238795325112867385, 1.000000000000000000, 0.9238795325112867385, 1.000000000000000000, 0.9238795325112867385, 1.000000000000000000, 0.9238795325112867385, 1.000000000000000000, 0.9238795325112867385, 1.000000000000000000, 0.9238795325112867385, 1.000000000000000000, 0.9238795325112867385, 1.000000000000000000, 0.9238795325112867385, 1.000000000000000000, 0.9238795325112867385, 1.000000000000000000, 0.9238795325112867385, 1.000000000000000000, 0.9238795325112867385, 1.000000000000000000, 0.9238795325112867385, 1.000000000000000000, 0.9238795325112867385, 1.000000000000000000, 0.9238795325112867385, 1.000000000000000000, 0.9238795325112867385, 1.000000000000000000, 0.9238795325112867385, 1.000000000000000000, 0.9238795325112867385, 1.000000000000000000, 0.9238795325112867385, 1.000000000000000000, 0.9238795325112867385, 1.000000000000000000, 0.9238795325112867385, 1.000000000000000000, 0.9238795325112867385, 1.000000000000000000, 0.9238795325112867385, 1.000000000000000000, 0.9238795325112867385, 1.000000000000000000, 0.9238795325112867385, 1.000000000000000000, 0.9238795325112867385, 1.000000000000000000, 0.9238795325112867385, 1.000000000000000000, 0.9238795325112867385, 1.000000000000000000, 0.9238795325112867385, 1.000000000000000000, 0.9238795325112867385, 1.000000000000000000, 0.9238795325112867385, 1.000000000000000000, 0.9238795325112867385, 1.000000000000000000, 0.9238795325112867385, 1.000000000000000000, 0.9238795325112867385, 1.000000000000000000, 0.9238795325112867385, 1.000000000000000000, 0.9238795325112867385, 1.000000000000000000, 0.9238795325112867385, 1.000000000000000000, 0.9238795325112867385, 1.000000000000000000, 0.9238795325112867385, 1.000000000000000000, 0.9238795325112867385, 1.000000000000000000, 0.9493985930367334625, 0.9660721903170175207) ) ) 
 REPRESENTATION_ITEM ( '' )  SURFACE ( )  );
#4699=CARTESIAN_POINT ( 'NONE',  ( -76.90625000204839523, 36.74823131438026280, 18.25176868561974786 ) ) ;
#4700=EDGE_CURVE ( 'NONE', #4769, #3987, #11233, .T. ) ;
#4707=CARTESIAN_POINT ( 'NONE',  ( -71.46875000204838102, 80.81189881250000440, -1.580522963032174394E-15 ) ) ;
#4710=VECTOR ( 'NONE', #1487, 1000.000000000000000 ) ;
#4711=EDGE_LOOP ( 'NONE', ( #4507, #11727, #4590, #8325 ) ) ;
#4714=LINE ( 'NONE', #2743, #5873 ) ;
#4717=CARTESIAN_POINT ( 'NONE',  ( 39.99999999999999289, 55.00000000000000000, 0.000000000000000000 ) ) ;
#4722=CARTESIAN_POINT ( 'NONE',  ( -15.00000000000000355, 5.000000000000000000, -29.99999999999999289 ) ) ;
#4730=CYLINDRICAL_SURFACE ( 'NONE', #9759, 24.99999999999999645 ) ;
#4732=CARTESIAN_POINT ( 'NONE',  ( -73.15625000204838102, 80.81189881250000440, -1.580522963032174394E-15 ) ) ;
#4735=CARTESIAN_POINT ( 'NONE',  ( -78.50000000204840944, 44.30836144126053000, 25.81189881250000795 ) ) ;
#4736=ORIENTED_EDGE ( 'NONE', *, *, #10695, .F. ) ;
#4737=( NAMED_UNIT ( * ) PLANE_ANGLE_UNIT ( ) SI_UNIT ( $, .RADIAN. ) );
#4738=AXIS2_PLACEMENT_3D ( 'NONE', #6164, #8011, #1383 ) ;
#4741=DIRECTION ( 'NONE',  ( 1.000000000000000000, 0.000000000000000000, 0.000000000000000000 ) ) ;
#4742=EDGE_CURVE ( 'NONE', #7798, #10526, #1299, .T. ) ;
#4745=AXIS2_PLACEMENT_3D ( 'NONE', #8396, #4806, #3780 ) ;
#4746=VERTEX_POINT ( 'NONE', #5752 ) ;
#4754=CARTESIAN_POINT ( 'NONE',  ( -15.00000000000000000, -24.99999999999999645, 10.00000000000000000 ) ) ;
#4760=CARTESIAN_POINT ( 'NONE',  ( -78.87500000204838102, 80.81189881250001861, 10.69163855873948599 ) ) ;
#4761=CARTESIAN_POINT ( 'NONE',  ( -15.00000000000000000, -30.00000000000000000, 10.00000000000000000 ) ) ;
#4765=CARTESIAN_POINT ( 'NONE',  ( -72.96875000204838102, 80.81189881250000440, -1.580522963032174394E-15 ) ) ;
#4769=VERTEX_POINT ( 'NONE', #93 ) ;
#4794=CARTESIAN_POINT ( 'NONE',  ( -0.8657091724475090011, 65.44905221436334841, -22.71165102530780899 ) ) ;
#4797=CARTESIAN_POINT ( 'NONE',  ( -71.46875000204838102, 80.81189881250000440, -1.580522963032174394E-15 ) ) ;
#4798=ORIENTED_EDGE ( 'NONE', *, *, #7702, .F. ) ;
#4799=CARTESIAN_POINT ( 'NONE',  ( 16.14987959356399472, 72.61399012904941230, -17.75150298415823258 ) ) ;
#4806=DIRECTION ( 'NONE',  ( -1.000000000000000000, -0.000000000000000000, -0.000000000000000000 ) ) ;
#4808=AXIS2_PLACEMENT_3D ( 'NONE', #5231, #8878, #7094 ) ;
#4810=CARTESIAN_POINT ( 'NONE',  ( -71.84302369010728739, 76.88501343918500197, 12.63531067400213104 ) ) ;
#4820=ADVANCED_FACE ( 'NONE', ( #8498 ), #278, .F. ) ;
#4821=DIRECTION ( 'NONE',  ( 1.000000000000000000, 0.000000000000000000, 0.000000000000000000 ) ) ;
#4825=CARTESIAN_POINT ( 'NONE',  ( -75.78125000204839523, 73.25176868561975141, 18.25176868561974075 ) ) ;
#4828=LINE ( 'NONE', #1996, #4435 ) ;
#4831=ORIENTED_EDGE ( 'NONE', *, *, #3960, .T. ) ;
#4842=CARTESIAN_POINT ( 'NONE',  ( -72.12500000000007105, 79.99999999999987210, -1.530808498934183830E-15 ) ) ;
#4856=PLANE ( 'NONE',  #11216 ) ;
#4857=CARTESIAN_POINT ( 'NONE',  ( -22.24057001764307984, 77.42300265451373775, 11.08010208964972954 ) ) ;
#4860=CARTESIAN_POINT ( 'NONE',  ( -73.15625000204839523, 73.25176868561975141, -18.25176868561974430 ) ) ;
#4862=CARTESIAN_POINT ( 'NONE',  ( 18.44309544900626463, 74.35063009805416812, -15.88073011970089432 ) ) ;
#4866=PLANE ( 'NONE',  #7979 ) ;
#4869=CARTESIAN_POINT ( 'NONE',  ( -73.43750000000000000, 72.67766952966368876, 17.67766952966368521 ) ) ;
#4876=DIRECTION ( 'NONE',  ( 1.000000000000000000, 0.000000000000000000, 0.000000000000000000 ) ) ;
#4877=ORIENTED_EDGE ( 'NONE', *, *, #10174, .F. ) ;
#4878=DIRECTION ( 'NONE',  ( 0.000000000000000000, 0.000000000000000000, -1.000000000000000000 ) ) ;
#4879=CARTESIAN_POINT ( 'NONE',  ( -78.50000000204842365, 29.18810118750000981, 10.69163855873950020 ) ) ;
#4886=CARTESIAN_POINT ( 'NONE',  ( -77.84375000409677625, 30.00000000000001421, 10.35533905932739174 ) ) ;
#4887=ORIENTED_EDGE ( 'NONE', *, *, #6623, .F. ) ;
#4892=VERTEX_POINT ( 'NONE', #5201 ) ;
#4900=ADVANCED_FACE ( 'NONE', ( #11353 ), #1480, .T. ) ;
#4901=ORIENTED_EDGE ( 'NONE', *, *, #8771, .T. ) ;
#4905=CARTESIAN_POINT ( 'NONE',  ( -77.28125000000004263, 30.00000000000009948, -10.35533905932734378 ) ) ;
#4919=CARTESIAN_POINT ( 'NONE',  ( -73.25000000204839523, 65.69163855873948421, -25.81189881250000440 ) ) ;
#4921=CARTESIAN_POINT ( 'NONE',  ( 22.23357492888157694, 77.41719160602768568, -11.09194826675321366 ) ) ;
#4926=CYLINDRICAL_SURFACE ( 'NONE', #4745, 24.99999999999999645 ) ;
#4929=CARTESIAN_POINT ( 'NONE',  ( -77.93750000000000000, 72.67766952966368876, 17.67766952966368521 ) ) ;
#4941=CARTESIAN_POINT ( 'NONE',  ( -76.34375000204839523, 73.25176868561975141, -18.25176868561974430 ) ) ;
#4942=ORIENTED_EDGE ( 'NONE', *, *, #1693, .T. ) ;
#4945=CARTESIAN_POINT ( 'NONE',  ( -72.40625000204839523, 36.74823131438026280, 18.25176868561974786 ) ) ;
#4951=CARTESIAN_POINT ( 'NONE',  ( 0.000000000000000000, -24.99999999999999645, 0.000000000000000000 ) ) ;
#4952=FACE_OUTER_BOUND ( 'NONE', #2652, .T. ) ;
#4962=VERTEX_POINT ( 'NONE', #6283 ) ;
#4975=CARTESIAN_POINT ( 'NONE',  ( -78.68750000204839523, 65.69163855873949842, 25.81189881250000084 ) ) ;
#4976=CARTESIAN_POINT ( 'NONE',  ( -24.25189443604024575, 79.11314215675321293, 6.649975675490534144 ) ) ;
#4980=CARTESIAN_POINT ( 'NONE',  ( -72.21875000204838102, 29.18810118750000271, 4.741568889096522788E-15 ) ) ;
#4990=CARTESIAN_POINT ( 'NONE',  ( -77.00000000000000000, 55.00000000000000000, -24.99999999999999645 ) ) ;
#4996=VECTOR ( 'NONE', #1151, 1000.000000000000000 ) ;
#4997=FACE_OUTER_BOUND ( 'NONE', #5206, .T. ) ;
#5001=CARTESIAN_POINT ( 'NONE',  ( 18.41311296310942325, 74.28344047684244345, -10.65941174978863337 ) ) ;
#5002=AXIS2_PLACEMENT_3D ( 'NONE', #4717, #1576, #2414 ) ;
#5003=CARTESIAN_POINT ( 'NONE',  ( -75.59375000204839523, 36.74823131438026280, 18.25176868561974786 ) ) ;
#5008=CARTESIAN_POINT ( 'NONE',  ( -72.59375000204838102, 55.00000000000000000, 25.81189881249999729 ) ) ;
#5031=FACE_OUTER_BOUND ( 'NONE', #7082, .T. ) ;
#5037=CARTESIAN_POINT ( 'NONE',  ( -78.21875000204839523, 29.18810118750000271, 4.741568889096522788E-15 ) ) ;
#5038=CARTESIAN_POINT ( 'NONE',  ( -21.38022012555706652, 76.71392452634511017, 12.39514039398179968 ) ) ;
#5041=CARTESIAN_POINT ( 'NONE',  ( -76.71875000409679046, 65.35533905932737753, 24.99999999999999645 ) ) ;
#5048=CARTESIAN_POINT ( 'NONE',  ( -73.90625000000007105, 65.35533905932732068, -24.99999999999986500 ) ) ;
#5051=CARTESIAN_POINT ( 'NONE',  ( -76.25000000000000000, 55.00000000000000000, 24.99999999999999645 ) ) ;
#5054=ORIENTED_EDGE ( 'NONE', *, *, #3285, .F. ) ;
#5057=CARTESIAN_POINT ( 'NONE',  ( -71.18677368791114191, 77.11938847399009944, 12.77062708069394503 ) ) ;
#5060=CARTESIAN_POINT ( 'NONE',  ( -4.067038661182964928E-21, 64.99605696851786263, 19.59792961213366169 ) ) ;
#5062=ORIENTED_EDGE ( 'NONE', *, *, #10409, .T. ) ;
#5063=VECTOR ( 'NONE', #8132, 1000.000000000000000 ) ;
#5064=CARTESIAN_POINT ( 'NONE',  ( -72.96875000204838102, 80.81189881250000440, -1.580522963032174394E-15 ) ) ;
#5065=EDGE_CURVE ( 'NONE', #6710, #494, #9080, .T. ) ;
#5079=CARTESIAN_POINT ( 'NONE',  ( 0.000000000000000000, -30.00000000000000000, -5.000000000000000000 ) ) ;
#5085=VECTOR ( 'NONE', #8305, 1000.000000000000000 ) ;
#5092=CARTESIAN_POINT ( 'NONE',  ( -75.96875000204839523, 80.81189881250000440, -1.580522963032174394E-15 ) ) ;
#5093=( BOUNDED_CURVE ( )  B_SPLINE_CURVE ( 2, ( #10431, #11443, #9545, #3979, #3194, #6866, #4213, #433, #1213, #9659, #7696, #4879, #8529, #11506, #6803, #3314, #7636, #11268, #493, #6981, #3079, #7876, #10490, #5972, #6750, #10378, #9608, #6925, #9483, #2173, #5842, #11329, #5902, #1272, #4941, #8598, #2355, #2233, #373, #6024, #3137, #1341, #5003, #8653, #1457, #5120, #7158, #7043, #8046, #1512, #1625, #10665, #722, #7932, #8108, #2474, #7218, #11744, #10844, #6317, #6261, #5570, #3547, #2594, #6140, #9836, #2651, #9716, #9949, #1005, #5176, #9004, #1902, #8946, #8831, #11687, #9217, #4665, #11061, #612, #8317, #665, #2535, #98, #3493, #4335, #7986 ),
 .UNSPECIFIED., .F., .T. ) 
 B_SPLINE_CURVE_WITH_KNOTS ( ( 3, 2, 2, 2, 2, 2, 2, 2, 2, 2, 2, 2, 2, 2, 2, 2, 2, 2, 2, 2, 2, 2, 2, 2, 2, 2, 2, 2, 2, 2, 2, 2, 2, 2, 2, 2, 2, 2, 2, 2, 2, 2, 2, 3 ),
 ( 0.000000000000000000, 0.02083333333333333218, 0.04166666666666666435, 0.06250000000000000000, 0.08333333333333332871, 0.1041666666666666713, 0.1250000000000000000, 0.1458333333333333426, 0.1666666666666666574, 0.1875000000000000000, 0.2083333333333333426, 0.2291666666666666297, 0.2500000000000000000, 0.2708333333333333148, 0.2916666666666666852, 0.3125000000000000000, 0.3333333333333333148, 0.3541666666666666852, 0.3750000000000000000, 0.3958333333333333148, 0.4166666666666666852, 0.4375000000000000000, 0.4583333333333332593, 0.4791666666666666852, 0.5000000000000000000, 0.5208333333333333703, 0.5416666666666666297, 0.5625000000000000000, 0.5833333333333333703, 0.6041666666666666297, 0.6250000000000000000, 0.6458333333333333703, 0.6666666666666666297, 0.6875000000000000000, 0.7083333333333333703, 0.7291666666666666297, 0.7500000000000000000, 0.7708333333333333703, 0.7916666666666666297, 0.8125000000000000000, 0.8333333333333333703, 0.8541666666666667407, 0.8750000000000000000, 0.8888490471511721891 ),
 .UNSPECIFIED. ) 
 CURVE ( )  GEOMETRIC_REPRESENTATION_ITEM ( )  RATIONAL_B_SPLINE_CURVE ( ( 1.000000000000000000, 0.9238795325112867385, 1.000000000000000000, 0.9238795325112867385, 1.000000000000000000, 0.9238795325112867385, 1.000000000000000000, 0.9238795325112867385, 1.000000000000000000, 0.9238795325112867385, 1.000000000000000000, 0.9238795325112867385, 1.000000000000000000, 0.9238795325112867385, 1.000000000000000000, 0.9238795325112867385, 1.000000000000000000, 0.9238795325112867385, 1.000000000000000000, 0.9238795325112867385, 1.000000000000000000, 0.9238795325112867385, 1.000000000000000000, 0.9238795325112867385, 1.000000000000000000, 0.9238795325112867385, 1.000000000000000000, 0.9238795325112867385, 1.000000000000000000, 0.9238795325112867385, 1.000000000000000000, 0.9238795325112867385, 1.000000000000000000, 0.9238795325112867385, 1.000000000000000000, 0.9238795325112867385, 1.000000000000000000, 0.9238795325112867385, 1.000000000000000000, 0.9238795325112867385, 1.000000000000000000, 0.9238795325112867385, 1.000000000000000000, 0.9238795325112867385, 1.000000000000000000, 0.9238795325112867385, 1.000000000000000000, 0.9238795325112867385, 1.000000000000000000, 0.9238795325112867385, 1.000000000000000000, 0.9238795325112867385, 1.000000000000000000, 0.9238795325112867385, 1.000000000000000000, 0.9238795325112867385, 1.000000000000000000, 0.9238795325112867385, 1.000000000000000000, 0.9238795325112867385, 1.000000000000000000, 0.9238795325112867385, 1.000000000000000000, 0.9238795325112867385, 1.000000000000000000, 0.9238795325112867385, 1.000000000000000000, 0.9238795325112867385, 1.000000000000000000, 0.9238795325112867385, 1.000000000000000000, 0.9238795325112867385, 1.000000000000000000, 0.9238795325112867385, 1.000000000000000000, 0.9238795325112867385, 1.000000000000000000, 0.9238795325112867385, 1.000000000000000000, 0.9238795325112867385, 1.000000000000000000, 0.9238795325112867385, 1.000000000000000000, 0.9238795325112867385, 1.000000000000000000, 0.9493985947158180005, 0.9660721892104719988 ) ) 
 REPRESENTATION_ITEM ( '' )  );
#5094=CARTESIAN_POINT ( 'NONE',  ( -21.60181664749086039, 76.89598700960922883, 12.07086080051332644 ) ) ;
#5098=CARTESIAN_POINT ( 'NONE',  ( -73.43750000409677625, 37.32233047033631124, 17.67766952966369232 ) ) ;
#5100=EDGE_LOOP ( 'NONE', ( #2877, #1287, #6475, #7057 ) ) ;
#5103=CARTESIAN_POINT ( 'NONE',  ( -75.50000000000001421, 54.99999999999944578, -24.99999999999999645 ) ) ;
#5105=CARTESIAN_POINT ( 'NONE',  ( -73.81250000000008527, 72.67766952966360350, -17.67766952966359639 ) ) ;
#5109=CARTESIAN_POINT ( 'NONE',  ( -74.46875000000000000, 30.00000000000001421, 10.35533905932739174 ) ) ;
#5116=( NAMED_UNIT ( * ) PLANE_ANGLE_UNIT ( ) SI_UNIT ( $, .RADIAN. ) );
#5117=VERTEX_POINT ( 'NONE', #11823 ) ;
#5118=CARTESIAN_POINT ( 'NONE',  ( 5.688665219163724807, 66.14467445454752692, -18.96884555856732035 ) ) ;
#5119=AXIS2_PLACEMENT_3D ( 'NONE', #2457, #1609, #5276 ) ;
#5120=CARTESIAN_POINT ( 'NONE',  ( -75.31250000204839523, 29.18810118750000626, -10.69163855873949132 ) ) ;
#5124=CARTESIAN_POINT ( 'NONE',  ( 9.999999999999994671, 0.000000000000000000, 10.00000000000000000 ) ) ;
#5125=CARTESIAN_POINT ( 'NONE',  ( -75.50000000409677625, 80.00000000000000000, -1.530808498934191324E-15 ) ) ;
#5128=STYLED_ITEM ( 'NONE', ( #7177 ), #9980 ) ;
#5136=CARTESIAN_POINT ( 'NONE',  ( -74.37500000204838102, 65.69163855873949842, 25.81189881250000440 ) ) ;
#5139=DIRECTION ( 'NONE',  ( 0.000000000000000000, 0.000000000000000000, 1.000000000000000000 ) ) ;
#5149=CARTESIAN_POINT ( 'NONE',  ( -78.78125000204839523, 73.25176868561975141, 18.25176868561974075 ) ) ;
#5150=FACE_OUTER_BOUND ( 'NONE', #6292, .T. ) ;
#5153=CARTESIAN_POINT ( 'NONE',  ( -75.40625000409677625, 80.00000000000001421, 10.35533905932737397 ) ) ;
#5154=CARTESIAN_POINT ( 'NONE',  ( -15.00000000000000355, 5.000000000000000000, -29.99999999999999289 ) ) ;
#5163=CARTESIAN_POINT ( 'NONE',  ( -78.21875000204839523, 36.74823131438024859, -18.25176868561973720 ) ) ;
#5165=VECTOR ( 'NONE', #585, 1000.000000000000000 ) ;
#5172=CYLINDRICAL_SURFACE ( 'NONE', #6707, 24.99999999999999645 ) ;
#5175=CARTESIAN_POINT ( 'NONE',  ( 20.06119547431871908, 75.62460108169236150, -7.685737028377098490 ) ) ;
#5176=CARTESIAN_POINT ( 'NONE',  ( -72.96875000204838102, 73.25176868561975141, 18.25176868561974075 ) ) ;
#5177=EDGE_LOOP ( 'NONE', ( #11401, #7432, #7136, #2356 ) ) ;
#5185=ADVANCED_FACE ( 'NONE', ( #6342, #9973 ), #6699, .F. ) ;
#5186=VECTOR ( 'NONE', #1691, 1000.000000000000000 ) ;
#5194=CARTESIAN_POINT ( 'NONE',  ( -78.87500000204838102, 65.69163855873949842, 25.81189881250000440 ) ) ;
#5201=CARTESIAN_POINT ( 'NONE',  ( 14.99999999999999645, -30.00000000000000000, 10.00000000000000000 ) ) ;
#5206=EDGE_LOOP ( 'NONE', ( #2449, #10266, #3809, #5054 ) ) ;
#5213=ORIENTED_EDGE ( 'NONE', *, *, #4284, .F. ) ;
#5214=CARTESIAN_POINT ( 'NONE',  ( -73.15625000409677625, 30.00000000000000355, -10.35533905932738108 ) ) ;
#5223=DIRECTION ( 'NONE',  ( 0.000000000000000000, 0.000000000000000000, -1.000000000000000000 ) ) ;
#5224=EDGE_CURVE ( 'NONE', #7962, #7402, #1015, .T. ) ;
#5227=CARTESIAN_POINT ( 'NONE',  ( -75.40625000204838102, 29.18810118750000271, 4.741568889096522788E-15 ) ) ;
#5231=CARTESIAN_POINT ( 'NONE',  ( -80.00000000000000000, 55.00000000000000000, 0.000000000000000000 ) ) ;
#5237=CARTESIAN_POINT ( 'NONE',  ( 21.03141440724603228, 76.42803413576605465, 5.034331618923938656 ) ) ;
#5241=CARTESIAN_POINT ( 'NONE',  ( 14.99999999999999645, -30.00000000000000000, 10.00000000000000000 ) ) ;
#5254=CARTESIAN_POINT ( 'NONE',  ( -77.37500000204838102, 65.69163855873949842, 25.81189881250000440 ) ) ;
#5255=VERTEX_POINT ( 'NONE', #385 ) ;
#5265=DIRECTION ( 'NONE',  ( -1.000000000000000000, -0.000000000000000000, -0.000000000000000000 ) ) ;
#5269=ORIENTED_EDGE ( 'NONE', *, *, #6814, .F. ) ;
#5270=CARTESIAN_POINT ( 'NONE',  ( -75.68750000409677625, 72.67766952966368876, -17.67766952966368876 ) ) ;
#5274=ORIENTED_EDGE ( 'NONE', *, *, #4187, .T. ) ;
#5276=DIRECTION ( 'NONE',  ( 0.000000000000000000, 0.000000000000000000, -1.000000000000000000 ) ) ;
#5280=CARTESIAN_POINT ( 'NONE',  ( -75.96875000204839523, 73.25176868561975141, 18.25176868561974075 ) ) ;
#5293=AXIS2_PLACEMENT_3D ( 'NONE', #2109, #4876, #8526 ) ;
#5295=ADVANCED_FACE ( 'NONE', ( #3147 ), #5913, .T. ) ;
#5309=CARTESIAN_POINT ( 'NONE',  ( -79.34375000204839523, 73.25176868561975141, -18.25176868561974430 ) ) ;
#5316=ADVANCED_FACE ( 'NONE', ( #4271, #1510 ), #5172, .T. ) ;
#5325=APPLICATION_CONTEXT ( 'automotive_design' ) ;
#5327=ORIENTED_EDGE ( 'NONE', *, *, #5224, .T. ) ;
#5335=ADVANCED_FACE ( 'NONE', ( #4952 ), #9354, .F. ) ;
#5337=ORIENTED_EDGE ( 'NONE', *, *, #9466, .F. ) ;
#5340=EDGE_CURVE ( 'NONE', #3514, #9870, #7573, .T. ) ;
#5341=CARTESIAN_POINT ( 'NONE',  ( -77.18750000204838102, 44.30836144126053000, 25.81189881250000795 ) ) ;
#5344=CARTESIAN_POINT ( 'NONE',  ( 0.000000000000000000, 110.0000000000000000, 27.53333900685068869 ) ) ;
#5345=ORIENTED_EDGE ( 'NONE', *, *, #5790, .T. ) ;
#5349=CYLINDRICAL_SURFACE ( 'NONE', #592, 5.249999999999998224 ) ;
#5366=EDGE_LOOP ( 'NONE', ( #6302, #5984, #7721, #7053 ) ) ;
#5368=CARTESIAN_POINT ( 'NONE',  ( -75.03125000204838102, 55.00000000000000000, -25.81189881249999729 ) ) ;
#5373=( NAMED_UNIT ( * ) PLANE_ANGLE_UNIT ( ) SI_UNIT ( $, .RADIAN. ) );
#5385=CARTESIAN_POINT ( 'NONE',  ( -75.68750000000005684, 37.32233047033638940, -17.67766952966360705 ) ) ;
#5387=ORIENTED_EDGE ( 'NONE', *, *, #2723, .T. ) ;
#5388=CARTESIAN_POINT ( 'NONE',  ( -71.09375000409677625, 80.00000000000001421, -10.35533905932737753 ) ) ;
#5390=CARTESIAN_POINT ( 'NONE',  ( 39.99999999999999289, 55.00000000000000000, -24.99999999999999645 ) ) ;
#5395=DIRECTION ( 'NONE',  ( 0.000000000000000000, 1.000000000000000000, 0.000000000000000000 ) ) ;
#5399=CARTESIAN_POINT ( 'NONE',  ( -74.28125000204838102, 55.00000000000000000, 25.81189881249999729 ) ) ;
#5403=CARTESIAN_POINT ( 'NONE',  ( -75.78125000204839523, 73.25176868561975141, 18.25176868561974075 ) ) ;
#5411=VERTEX_POINT ( 'NONE', #2269 ) ;
#5425=CARTESIAN_POINT ( 'NONE',  ( -79.15625000204839523, 73.25176868561975141, -18.25176868561974430 ) ) ;
#5431=EDGE_CURVE ( 'NONE', #896, #7402, #3175, .T. ) ;
#5435=ORIENTED_EDGE ( 'NONE', *, *, #1143, .T. ) ;
#5440=DIRECTION ( 'NONE',  ( 0.000000000000000000, 0.000000000000000000, 1.000000000000000000 ) ) ;
#5444=CARTESIAN_POINT ( 'NONE',  ( -76.62500000000005684, 79.99999999999991473, -1.530808498934185605E-15 ) ) ;
#5450=EDGE_LOOP ( 'NONE', ( #8877, #7543, #5345, #4625 ) ) ;
#5454=CARTESIAN_POINT ( 'NONE',  ( -2.149629781808683138, 65.58267949266357277, -22.64980306772420349 ) ) ;
#5458=CARTESIAN_POINT ( 'NONE',  ( -76.62500000204839523, 29.18810118750000626, -10.69163855873949309 ) ) ;
#5459=ORIENTED_EDGE ( 'NONE', *, *, #5224, .F. ) ;
#5460=CARTESIAN_POINT ( 'NONE',  ( 12.37746768708380074, 69.98505844884790861, 20.01803919467661430 ) ) ;
#5463=CARTESIAN_POINT ( 'NONE',  ( -79.25000000000000000, 55.00000000000000000, 24.99999999999999645 ) ) ;
#5469=( BOUNDED_CURVE ( )  B_SPLINE_CURVE ( 2, ( #6822, #5919, #8615, #270, #3933, #4062, #6642, #11346, #214 ),
 .UNSPECIFIED., .F., .T. ) 
 B_SPLINE_CURVE_WITH_KNOTS ( ( 3, 2, 2, 2, 3 ),
 ( 0.2500000000000002220, 0.2708333333333335369, 0.2916666666666669627, 0.3125000000000002776, 0.3333333333333335924 ),
 .UNSPECIFIED. ) 
 CURVE ( )  GEOMETRIC_REPRESENTATION_ITEM ( )  RATIONAL_B_SPLINE_CURVE ( ( 0.9999999999999992228, 0.9238795325112875156, 1.000000000000000000, 0.9238795325112867385, 1.000000000000000000, 0.9238795325112867385, 1.000000000000000000, 0.9238795325112857393, 1.000000000000001110 ) ) 
 REPRESENTATION_ITEM ( '' )  );
#5472=CARTESIAN_POINT ( 'NONE',  ( -3.965853256712214225, 65.56424026801020943, -19.29796592139343758 ) ) ;
#5473=AXIS2_PLACEMENT_3D ( 'NONE', #10631, #2262, #8017 ) ;
#5480=CARTESIAN_POINT ( 'NONE',  ( -73.25000000204838102, 80.81189881250001861, -10.69163855873949132 ) ) ;
#5482=EDGE_CURVE ( 'NONE', #9843, #388, #1550, .T. ) ;
#5483=ORIENTED_EDGE ( 'NONE', *, *, #8211, .F. ) ;
#5487=VERTEX_POINT ( 'NONE', #6062 ) ;
#5497=AXIS2_PLACEMENT_3D ( 'NONE', #4951, #6578, #7648 ) ;
#5499=DIRECTION ( 'NONE',  ( 0.000000000000000000, 0.000000000000000000, -1.000000000000000000 ) ) ;
#5500=EDGE_CURVE ( 'NONE', #10858, #7962, #4252, .T. ) ;
#5506=VECTOR ( 'NONE', #10965, 1000.000000000000000 ) ;
#5513=CARTESIAN_POINT ( 'NONE',  ( -18.39575369641156399, 74.32255031325632899, -15.87762562984429415 ) ) ;
#5517=CARTESIAN_POINT ( 'NONE',  ( -76.06250000204840944, 80.81189881250001861, -10.69163855873949132 ) ) ;
#5519=CARTESIAN_POINT ( 'NONE',  ( 11.01771772720809572, 69.13422207321994506, 20.62759405020127801 ) ) ;
#5525=CARTESIAN_POINT ( 'NONE',  ( -79.90625000000000000, 65.35533905932737753, -24.99999999999999645 ) ) ;
#5532=CARTESIAN_POINT ( 'NONE',  ( -20.85448682672772946, 76.28028968605049442, -5.762572995040112112 ) ) ;
#5537=CARTESIAN_POINT ( 'NONE',  ( -74.18750000409677625, 72.67766952966368876, -17.67766952966368876 ) ) ;
#5541=CARTESIAN_POINT ( 'NONE',  ( -78.12500000204838102, 29.18810118750000626, -10.69163855873949309 ) ) ;
#5544=ORIENTED_EDGE ( 'NONE', *, *, #3019, .T. ) ;
#5550=APPLICATION_CONTEXT ( 'automotive_design' ) ;
#5558=DIRECTION ( 'NONE',  ( 0.000000000000000000, 0.000000000000000000, 1.000000000000000000 ) ) ;
#5562=DIRECTION ( 'NONE',  ( 0.000000000000000000, 0.000000000000000000, -1.000000000000000000 ) ) ;
#5570=CARTESIAN_POINT ( 'NONE',  ( -73.81250000204839523, 29.18810118750000626, -10.69163855873949132 ) ) ;
#5574=CARTESIAN_POINT ( 'NONE',  ( -23.65491598197041156, 78.60782538777030481, -8.235832699802983825 ) ) ;
#5577=ORIENTED_EDGE ( 'NONE', *, *, #6690, .F. ) ;
#5578=ADVANCED_FACE ( 'NONE', ( #3405 ), #3344, .F. ) ;
#5584=FACE_OUTER_BOUND ( 'NONE', #940, .T. ) ;
#5594=CARTESIAN_POINT ( 'NONE',  ( -79.15625000000000000, 44.64466094067262958, 25.00000000000001066 ) ) ;
#5601=CARTESIAN_POINT ( 'NONE',  ( -7.621884045487905546, 66.99230996961183848, -18.44821524278371427 ) ) ;
#5605=LINE ( 'NONE', #11208, #766 ) ;
#5608=CARTESIAN_POINT ( 'NONE',  ( -71.65625000204838102, 80.81189881250000440, -1.580522963032174394E-15 ) ) ;
#5638=CARTESIAN_POINT ( 'NONE',  ( -71.59560441993426139, 80.81189881250000440, 6.916273537586018705 ) ) ;
#5644=CARTESIAN_POINT ( 'NONE',  ( -15.00000000000000000, -24.99999999999999645, -10.00000000000000000 ) ) ;
#5648=CARTESIAN_POINT ( 'NONE',  ( -78.59375000000001421, 44.64466094067260826, -24.99999999999998934 ) ) ;
#5652=EDGE_CURVE ( 'NONE', #9870, #7798, #2516, .T. ) ;
#5656=CARTESIAN_POINT ( 'NONE',  ( -21.03106668926508149, 76.42784099770780415, 4.997211433137191960 ) ) ;
#5657=CARTESIAN_POINT ( 'NONE',  ( 2.782474192756827142E-15, 65.42943686846950868, -22.72062601704910634 ) ) ;
#5660=EDGE_CURVE ( 'NONE', #6052, #847, #10447, .T. ) ;
#5661=DIRECTION ( 'NONE',  ( 1.000000000000000000, 0.000000000000000000, 0.000000000000000000 ) ) ;
#5665=CARTESIAN_POINT ( 'NONE',  ( -72.87500000204839523, 65.69163855873949842, 25.81189881250000440 ) ) ;
#5668=DIRECTION ( 'NONE',  ( -1.000000000000000000, -0.000000000000000000, -0.000000000000000000 ) ) ;
#5671=VERTEX_POINT ( 'NONE', #10507 ) ;
#5679=CARTESIAN_POINT ( 'NONE',  ( -73.25000000409677625, 30.00000000000000355, 4.592425496802573578E-15 ) ) ;
#5682=CARTESIAN_POINT ( 'NONE',  ( 39.99999999999999289, 55.00000000000000000, 0.000000000000000000 ) ) ;
#5694=ORIENTED_EDGE ( 'NONE', *, *, #2362, .F. ) ;
#5699=CARTESIAN_POINT ( 'NONE',  ( -19.95440955002869288, 75.55706508317430803, -14.23123435947546511 ) ) ;
#5703=CARTESIAN_POINT ( 'NONE',  ( -72.68750000204839523, 65.69163855873949842, 25.81189881250000440 ) ) ;
#5705=CARTESIAN_POINT ( 'NONE',  ( 25.23800105611221767, 79.95549307754095025, 1.714966265850949689 ) ) ;
#5708=EDGE_CURVE ( 'NONE', #1153, #3359, #2189, .T. ) ;
#5711=EDGE_CURVE ( 'NONE', #10129, #10562, #1356, .T. ) ;
#5714=CARTESIAN_POINT ( 'NONE',  ( -78.50000000000000000, 55.00000000000000000, -24.99999999999999645 ) ) ;
#5719=B_SPLINE_CURVE_WITH_KNOTS ( 'NONE', 3,
 ( #1793, #11739, #9944, #7213, #3662, #3488, #9053, #829, #7378, #4502, #7153, #11005, #2817, #1678, #5519, #5460, #10776, #2762, #11796, #9108, #6485, #888, #6423, #8155, #2589, #3602, #7267, #10897, #6372, #10112, #8938, #716, #4563, #4387, #3121, #7506, #9343, #5705, #9404, #8392, #2156, #3775, #3957, #1132, #6729, #1198, #8457, #7619, #107, #235, #8573, #6609, #4921, #3899, #4673, #2880, #10361, #5827, #4862, #7676, #4799, #2030, #10236, #352, #8326, #7562, #8512, #7443, #11186, #2999, #9465, #6668, #171, #2093, #5766, #10180 ),
 .UNSPECIFIED., .F., .F.,
 ( 4, 2, 2, 2, 2, 2, 2, 2, 2, 2, 2, 2, 2, 2, 2, 2, 2, 2, 2, 2, 2, 2, 2, 2, 2, 2, 2, 2, 2, 2, 2, 2, 2, 2, 2, 2, 2, 4 ),
 ( 0.07733197755222971648, 0.07860774102649789596, 0.07988350450076606157, 0.08243503144930242055, 0.08371079492357058616, 0.08498655839783876564, 0.08753808534637511074, 0.09008961229491145584, 0.09264113924344780093, 0.09774419314052049113, 0.09901995661478867061, 0.1002957200890568501, 0.1028472470375931952, 0.1053987739861295403, 0.1066745374603977198, 0.1079503009346658993, 0.1130533548317386588, 0.1143291183060068522, 0.1156048817802750456, 0.1181564087288114462, 0.1194321722030796395, 0.1207079356773478329, 0.1232594626258842058, 0.1245352261001523991, 0.1258109895744205786, 0.1283625165229569931, 0.1309140434714933798, 0.1321898069457616010, 0.1334655704200297666, 0.1385686243171025123, 0.1411201512656388712, 0.1436716782141752302, 0.1487747321112479759, 0.1500504955855161415, 0.1513262590597843626, 0.1538777860083207216, 0.1564293129568570806, 0.1589808399053934673 ),
 .UNSPECIFIED. ) ;
#5722=CARTESIAN_POINT ( 'NONE',  ( -12.86109194577659132, 70.12932790242416559, 15.98028952803886860 ) ) ;
#5725=PLANE ( 'NONE',  #1481 ) ;
#5727=CARTESIAN_POINT ( 'NONE',  ( -74.09375000409677625, 80.00000000000001421, -10.35533905932737753 ) ) ;
#5734=CARTESIAN_POINT ( 'NONE',  ( -15.00000000000000000, -30.00000000000000000, 10.00000000000000000 ) ) ;
#5736=CARTESIAN_POINT ( 'NONE',  ( -72.40625000204839523, 36.74823131438026280, 18.25176868561974786 ) ) ;
#5739=ORIENTED_EDGE ( 'NONE', *, *, #996, .F. ) ;
#5752=CARTESIAN_POINT ( 'NONE',  ( -74.37500000409677625, 55.00000000000000000, -24.99999999999999645 ) ) ;
#5756=ORIENTED_EDGE ( 'NONE', *, *, #11547, .F. ) ;
#5761=CARTESIAN_POINT ( 'NONE',  ( -25.03138265018328568, 79.77837991132803097, -3.428720668973124663 ) ) ;
#5764=CARTESIAN_POINT ( 'NONE',  ( -72.87500000204840944, 80.81189881250001861, 10.69163855873948599 ) ) ;
#5766=CARTESIAN_POINT ( 'NONE',  ( 0.8611532375456804056, 65.42943686846948026, -22.72062601704910278 ) ) ;
#5773=EDGE_LOOP ( 'NONE', ( #6687, #744, #5387, #11813 ) ) ;
#5782=CARTESIAN_POINT ( 'NONE',  ( -72.59375000000008527, 44.64466094067266511, -24.99999999999984723 ) ) ;
#5788=CARTESIAN_POINT ( 'NONE',  ( 36.99999999999999289, 55.00000000000000000, 0.000000000000000000 ) ) ;
#5790=EDGE_CURVE ( 'NONE', #6077, #5487, #8547, .T. ) ;
#5791=ORIENTED_EDGE ( 'NONE', *, *, #4460, .T. ) ;
#5794=CARTESIAN_POINT ( 'NONE',  ( -73.15625000204839523, 73.25176868561975141, -18.25176868561974430 ) ) ;
#5796=CARTESIAN_POINT ( 'NONE',  ( -79.25000000000000000, 55.00000000000000000, 24.99999999999999645 ) ) ;
#5799=CARTESIAN_POINT ( 'NONE',  ( -71.56250000204840944, 80.81189881250000440, -10.69163855873948954 ) ) ;
#5816=ORIENTED_EDGE ( 'NONE', *, *, #1242, .T. ) ;
#5819=FACE_OUTER_BOUND ( 'NONE', #5450, .T. ) ;
#5822=CARTESIAN_POINT ( 'NONE',  ( -25.29045292946807422, 80.00055243027901497, 0.3925393747600745553 ) ) ;
#5825=CARTESIAN_POINT ( 'NONE',  ( -78.59375000409679046, 80.00000000000001421, -10.35533905932737753 ) ) ;
#5827=CARTESIAN_POINT ( 'NONE',  ( 19.49008781870746176, 75.18049492239477161, -14.82407953042221038 ) ) ;
#5832=ORIENTED_EDGE ( 'NONE', *, *, #8564, .F. ) ;
#5833=CARTESIAN_POINT ( 'NONE',  ( -77.65625000000001421, 44.64466094067262958, 25.00000000000001066 ) ) ;
#5842=CARTESIAN_POINT ( 'NONE',  ( -76.71875000204839523, 36.74823131438024859, -18.25176868561973720 ) ) ;
#5843=ORIENTED_EDGE ( 'NONE', *, *, #426, .F. ) ;
#5845=CARTESIAN_POINT ( 'NONE',  ( -73.81250000204839523, 29.18810118750000981, 10.69163855873950020 ) ) ;
#5851=CARTESIAN_POINT ( 'NONE',  ( -78.03125000409679046, 44.64466094067260826, 24.99999999999998579 ) ) ;
#5853=CARTESIAN_POINT ( 'NONE',  ( -71.40810441781459872, 80.81189881250000440, 6.916273779317701376 ) ) ;
#5854=DIRECTION ( 'NONE',  ( 0.000000000000000000, 0.000000000000000000, 1.000000000000000000 ) ) ;
#5857=ORIENTED_EDGE ( 'NONE', *, *, #7203, .F. ) ;
#5861=CARTESIAN_POINT ( 'NONE',  ( 14.99999999999999645, 55.00000000000000000, 20.00000000000000000 ) ) ;
#5865=( BOUNDED_CURVE ( )  B_SPLINE_CURVE ( 2, ( #9872, #10766, #7144, #8988, #9214, #10224, #1961, #9153, #1899 ),
 .UNSPECIFIED., .F., .T. ) 
 B_SPLINE_CURVE_WITH_KNOTS ( ( 3, 2, 2, 2, 3 ),
 ( 0.000000000000000000, 0.02083333333333334952, 0.04166666666666669905, 0.06250000000000005551, 0.08333333333333339810 ),
 .UNSPECIFIED. ) 
 CURVE ( )  GEOMETRIC_REPRESENTATION_ITEM ( )  RATIONAL_B_SPLINE_CURVE ( ( 1.000000000000000000, 0.9238795325112867385, 1.000000000000000000, 0.9238795325112867385, 1.000000000000000000, 0.9238795325112867385, 1.000000000000000000, 0.9238795325112865164, 1.000000000000000222 ) ) 
 REPRESENTATION_ITEM ( '' )  );
#5869=CYLINDRICAL_SURFACE ( 'NONE', #1279, 24.99999999999999645 ) ;
#5873=VECTOR ( 'NONE', #2007, 1000.000000000000000 ) ;
#5874=DIRECTION ( 'NONE',  ( 0.000000000000000000, 0.000000000000000000, 1.000000000000000000 ) ) ;
#5877=CARTESIAN_POINT ( 'NONE',  ( -77.84375000204839523, 55.00000000000000000, -25.81189881249999729 ) ) ;
#5880=CARTESIAN_POINT ( 'NONE',  ( -71.93750000204838102, 44.30836144126050158, -25.81189881249999374 ) ) ;
#5887=CARTESIAN_POINT ( 'NONE',  ( -15.00000000000000355, 5.000000000000000000, 30.00000000000000711 ) ) ;
#5888=PLANE ( 'NONE',  #1683 ) ;
#5891=CARTESIAN_POINT ( 'NONE',  ( -72.78125000000002842, 30.00000000000000355, -10.35533905932738108 ) ) ;
#5894=ADVANCED_FACE ( 'NONE', ( #796 ), #4698, .F. ) ;
#5901=CARTESIAN_POINT ( 'NONE',  ( 15.84255450020419964, 72.28565062628483417, -13.62130773388284055 ) ) ;
#5902=CARTESIAN_POINT ( 'NONE',  ( -76.53125000204838102, 55.00000000000000000, -25.81189881249999729 ) ) ;
#5907=CARTESIAN_POINT ( 'NONE',  ( -75.31250000409677625, 72.67766952966368876, 17.67766952966368521 ) ) ;
#5908=CARTESIAN_POINT ( 'NONE',  ( 0.000000000000000000, -30.00000000000000000, -5.000000000000000000 ) ) ;
#5910=CARTESIAN_POINT ( 'NONE',  ( 14.99999999999999645, 5.000000000000000000, -19.99999999999999645 ) ) ;
#5911=ORIENTED_EDGE ( 'NONE', *, *, #10075, .F. ) ;
#5913=PLANE ( 'NONE',  #5931 ) ;
#5919=CARTESIAN_POINT ( 'NONE',  ( -76.53125000409679046, 44.64466094067255142, 24.99999999999992184 ) ) ;
#5931=AXIS2_PLACEMENT_3D ( 'NONE', #1570, #6816, #6761 ) ;
#5935=CYLINDRICAL_SURFACE ( 'NONE', #10778, 22.00000000000000000 ) ;
#5937=CARTESIAN_POINT ( 'NONE',  ( -77.18750000204839523, 65.69163855873949842, 25.81189881250000084 ) ) ;
#5942=CARTESIAN_POINT ( 'NONE',  ( -78.40625000409677625, 80.00000000000001421, 10.35533905932737397 ) ) ;
#5958=CARTESIAN_POINT ( 'NONE',  ( -77.18750000000000000, 37.32233047033631124, -17.67766952966368166 ) ) ;
#5960=CARTESIAN_POINT ( 'NONE',  ( 9.999999999999994671, -24.99999999999999645, 10.00000000000000000 ) ) ;
#5961=ORIENTED_EDGE ( 'NONE', *, *, #10757, .T. ) ;
#5969=ORIENTED_EDGE ( 'NONE', *, *, #10336, .F. ) ;
#5970=CARTESIAN_POINT ( 'NONE',  ( 20.05122251396076649, 75.61688920795575086, 7.685058149121978488 ) ) ;
#5971=CIRCLE ( 'NONE', #772, 5.000000000000000000 ) ;
#5972=CARTESIAN_POINT ( 'NONE',  ( -77.37500000204838102, 65.69163855873949842, 25.81189881250000084 ) ) ;
#5974=CARTESIAN_POINT ( 'NONE',  ( -74.65625000204839523, 73.25176868561975141, -18.25176868561974430 ) ) ;
#5984=ORIENTED_EDGE ( 'NONE', *, *, #9211, .T. ) ;
#6000=CARTESIAN_POINT ( 'NONE',  ( -78.40625000204839523, 36.74823131438026280, 18.25176868561974786 ) ) ;
#6002=CARTESIAN_POINT ( 'NONE',  ( -0.8575857771174034694, 65.42943686846950868, 22.72062601704910634 ) ) ;
#6005=CARTESIAN_POINT ( 'NONE',  ( -72.31250000409677625, 72.67766952966368876, 17.67766952966368521 ) ) ;
#6012=DIRECTION ( 'NONE',  ( -1.000000000000000000, 0.000000000000000000, 0.000000000000000000 ) ) ;
#6015=CARTESIAN_POINT ( 'NONE',  ( -74.37500000000000000, 30.00000000000000355, 4.592425496802573578E-15 ) ) ;
#6017=DIRECTION ( 'NONE',  ( 1.000000000000000000, -0.000000000000000000, -0.000000000000000000 ) ) ;
#6023=CARTESIAN_POINT ( 'NONE',  ( 21.71463995357127885, 77.00007676519764743, -0.7273169618903911893 ) ) ;
#6024=CARTESIAN_POINT ( 'NONE',  ( -75.87500000204838102, 65.69163855873949842, 25.81189881250000084 ) ) ;
#6044=EDGE_LOOP ( 'NONE', ( #7171, #3156, #4942, #4180 ) ) ;
#6052=VERTEX_POINT ( 'NONE', #10544 ) ;
#6056=CARTESIAN_POINT ( 'NONE',  ( -75.78125000204839523, 73.25176868561975141, 18.25176868561974075 ) ) ;
#6061=CARTESIAN_POINT ( 'NONE',  ( -74.00000000409677625, 80.00000000000000000, -1.530808498934191324E-15 ) ) ;
#6062=CARTESIAN_POINT ( 'NONE',  ( -80.00000000000000000, 55.00000000000000000, 22.00000000000000000 ) ) ;
#6070=CARTESIAN_POINT ( 'NONE',  ( -79.53125000204838102, 55.00000000000000000, -25.81189881249999729 ) ) ;
#6071=CARTESIAN_POINT ( 'NONE',  ( -74.84375000000000000, 65.35533905932737753, 24.99999999999999645 ) ) ;
#6077=VERTEX_POINT ( 'NONE', #3303 ) ;
#6081=CARTESIAN_POINT ( 'NONE',  ( 14.40112391949197779, 71.21751140778172839, 14.87572979763152681 ) ) ;
#6086=ADVANCED_FACE ( 'NONE', ( #2347 ), #655, .F. ) ;
#6087=LINE ( 'NONE', #8951, #9410 ) ;
#6088=LINE ( 'NONE', #6929, #8463 ) ;
#6102=ORIENTED_EDGE ( 'NONE', *, *, #10184, .F. ) ;
#6116=CARTESIAN_POINT ( 'NONE',  ( -72.96875000409677625, 44.64466094067260826, -24.99999999999998934 ) ) ;
#6129=CARTESIAN_POINT ( 'NONE',  ( -76.90625000204838102, 29.18810118750000271, 4.741568889096522788E-15 ) ) ;
#6140=CARTESIAN_POINT ( 'NONE',  ( -73.53125000204838102, 55.00000000000000000, -25.81189881249999729 ) ) ;
#6145=VECTOR ( 'NONE', #3707, 1000.000000000000000 ) ;
#6154=ORIENTED_EDGE ( 'NONE', *, *, #9135, .F. ) ;
#6158=CARTESIAN_POINT ( 'NONE',  ( -76.62500000204839523, 44.30836144126050158, -25.81189881249999374 ) ) ;
#6161=ORIENTED_EDGE ( 'NONE', *, *, #2392, .F. ) ;
#6164=CARTESIAN_POINT ( 'NONE',  ( 0.000000000000000000, 0.000000000000000000, 0.000000000000000000 ) ) ;
#6173=PLANE ( 'NONE',  #5473 ) ;
#6175=CARTESIAN_POINT ( 'NONE',  ( 39.99999999999999289, 55.00000000000000000, 0.000000000000000000 ) ) ;
#6179=DIRECTION ( 'NONE',  ( 0.000000000000000000, 0.000000000000000000, -1.000000000000000000 ) ) ;
#6180=CARTESIAN_POINT ( 'NONE',  ( -15.00000000000000000, -24.99999999999999645, 10.00000000000000000 ) ) ;
#6192=CARTESIAN_POINT ( 'NONE',  ( -75.78125000204838102, 55.00000000000000000, 25.81189881249999729 ) ) ;
#6212=FACE_OUTER_BOUND ( 'NONE', #1870, .T. ) ;
#6216=CARTESIAN_POINT ( 'NONE',  ( -76.06250000204839523, 80.81189881250001861, 10.69163855873948599 ) ) ;
#6234=ORIENTED_EDGE ( 'NONE', *, *, #5482, .F. ) ;
#6235=CARTESIAN_POINT ( 'NONE',  ( -71.46875000409677625, 44.64466094067260826, -24.99999999999998934 ) ) ;
#6236=CARTESIAN_POINT ( 'NONE',  ( -15.00000000000000000, 55.00000000000000000, 20.00000000000000000 ) ) ;
#6249=CARTESIAN_POINT ( 'NONE',  ( -72.06435441788588037, 80.00000000000001421, 6.698726029249594482 ) ) ;
#6259=VECTOR ( 'NONE', #11166, 1000.000000000000000 ) ;
#6261=CARTESIAN_POINT ( 'NONE',  ( -73.90625000204838102, 29.18810118750000271, 4.741568889096522788E-15 ) ) ;
#6265=LINE ( 'NONE', #7991, #610 ) ;
#6282=FILL_AREA_STYLE ('',( #7064 ) ) ;
#6283=CARTESIAN_POINT ( 'NONE',  ( 14.99999999999999645, 5.000000000000000000, 30.00000000000000711 ) ) ;
#6292=EDGE_LOOP ( 'NONE', ( #9083, #502, #7922, #11618 ) ) ;
#6302=ORIENTED_EDGE ( 'NONE', *, *, #2580, .T. ) ;
#6305=CARTESIAN_POINT ( 'NONE',  ( -74.37500000204838102, 65.69163855873949842, 25.81189881250000440 ) ) ;
#6308=CARTESIAN_POINT ( 'NONE',  ( -76.43750000204839523, 44.30836144126050158, -25.81189881249999374 ) ) ;
#6313=CARTESIAN_POINT ( 'NONE',  ( -15.00000000000000000, 39.99999999999999289, 20.00000000000000000 ) ) ;
#6317=CARTESIAN_POINT ( 'NONE',  ( -74.00000000204838102, 29.18810118750000981, 10.69163855873950020 ) ) ;
#6329=DIRECTION ( 'NONE',  ( 0.000000000000000000, 0.000000000000000000, 1.000000000000000000 ) ) ;
#6330=ADVANCED_FACE ( 'NONE', ( #9036 ), #8307, .F. ) ;
#6333=ORIENTED_EDGE ( 'NONE', *, *, #7566, .T. ) ;
#6335=CARTESIAN_POINT ( 'NONE',  ( -78.68750000204838102, 44.30836144126053000, 25.81189881250000795 ) ) ;
#6342=FACE_BOUND ( 'NONE', #9069, .T. ) ;
#6352=ORIENTED_EDGE ( 'NONE', *, *, #6789, .T. ) ;
#6363=LINE ( 'NONE', #3651, #10285 ) ;
#6366=CARTESIAN_POINT ( 'NONE',  ( -78.50000000204840944, 29.18810118750000981, 10.69163855873950020 ) ) ;
#6370=CARTESIAN_POINT ( 'NONE',  ( -78.96875000204839523, 80.81189881250000440, -1.580522963032174394E-15 ) ) ;
#6372=CARTESIAN_POINT ( 'NONE',  ( 22.22529492952226704, 77.41112953092405746, 11.08543588549235182 ) ) ;
#6380=FACE_OUTER_BOUND ( 'NONE', #3840, .T. ) ;
#6382=CARTESIAN_POINT ( 'NONE',  ( -15.00000000000000355, 5.000000000000000000, -29.99999999999999289 ) ) ;
#6389=( BOUNDED_CURVE ( )  B_SPLINE_CURVE ( 2, ( #10071, #2053, #5537, #5727, #7398, #1933, #8474, #4695, #6441 ),
 .UNSPECIFIED., .F., .T. ) 
 B_SPLINE_CURVE_WITH_KNOTS ( ( 3, 2, 2, 2, 3 ),
 ( 0.5000000000000004441, 0.5208333333333338144, 0.5416666666666670737, 0.5625000000000004441, 0.5833333333333338144 ),
 .UNSPECIFIED. ) 
 CURVE ( )  GEOMETRIC_REPRESENTATION_ITEM ( )  RATIONAL_B_SPLINE_CURVE ( ( 0.9999999999999983347, 0.9238795325112884038, 1.000000000000000000, 0.9238795325112867385, 1.000000000000000000, 0.9238795325112867385, 1.000000000000000000, 0.9238795325112850731, 1.000000000000001554 ) ) 
 REPRESENTATION_ITEM ( '' )  );
#6390=CARTESIAN_POINT ( 'NONE',  ( -73.53125000204838102, 55.00000000000000000, -25.81189881249999729 ) ) ;
#6399=ORIENTED_EDGE ( 'NONE', *, *, #7701, .F. ) ;
#6404=CARTESIAN_POINT ( 'NONE',  ( 0.000000000000000000, -30.00000000000000000, 0.000000000000000000 ) ) ;
#6406=CARTESIAN_POINT ( 'NONE',  ( -70.93935441986302237, 79.99999999999998579, 6.698726263377742463 ) ) ;
#6411=EDGE_LOOP ( 'NONE', ( #3971, #104 ) ) ;
#6416=CARTESIAN_POINT ( 'NONE',  ( -8.886150220881933848, 67.92913895864731444, -21.40220125730746759 ) ) ;
#6417=B_SPLINE_CURVE_WITH_KNOTS ( 'NONE', 1,
 ( #9824, #6070 ),
 .UNSPECIFIED., .F., .F.,
 ( 2, 2 ),
 ( 0.000000000000000000, 1.000000000000000000 ),
 .UNSPECIFIED. ) ;
#6421=CARTESIAN_POINT ( 'NONE',  ( -76.53125000204839523, 36.74823131438024859, -18.25176868561973720 ) ) ;
#6422=ORIENTED_EDGE ( 'NONE', *, *, #5708, .T. ) ;
#6423=CARTESIAN_POINT ( 'NONE',  ( 18.68839539025461605, 74.55286672756655264, 15.58206179569618577 ) ) ;
#6426=CARTESIAN_POINT ( 'NONE',  ( -78.68750000000002842, 37.32233047033633966, -17.67766952966366034 ) ) ;
#6435=CARTESIAN_POINT ( 'NONE',  ( -20.82524276125487361, 76.25657222871954843, 5.681780444169967303 ) ) ;
#6441=CARTESIAN_POINT ( 'NONE',  ( -73.62500000409677625, 55.00000000000000000, 24.99999999999999645 ) ) ;
#6444=CARTESIAN_POINT ( 'NONE',  ( -78.03125000204839523, 36.74823131438024859, -18.25176868561973720 ) ) ;
#6458=EDGE_CURVE ( 'NONE', #7798, #11523, #9205, .T. ) ;
#6461=CARTESIAN_POINT ( 'NONE',  ( -73.62500000409677625, 55.00000000000000000, 24.99999999999999645 ) ) ;
#6466=CARTESIAN_POINT ( 'NONE',  ( 0.000000000000000000, -30.00000000000000000, 0.000000000000000000 ) ) ;
#6475=ORIENTED_EDGE ( 'NONE', *, *, #2866, .T. ) ;
#6477=CARTESIAN_POINT ( 'NONE',  ( 9.999999999999994671, 0.000000000000000000, -10.00000000000000000 ) ) ;
#6479=CARTESIAN_POINT ( 'NONE',  ( -73.06250000204840944, 80.81189881250001861, 10.69163855873948599 ) ) ;
#6483=CARTESIAN_POINT ( 'NONE',  ( -77.56250000204839523, 80.81189881250001861, -10.69163855873949132 ) ) ;
#6485=CARTESIAN_POINT ( 'NONE',  ( 17.86907162826477702, 73.91589606910815746, 16.34925201472697864 ) ) ;
#6489=FACE_OUTER_BOUND ( 'NONE', #4711, .T. ) ;
#6499=VECTOR ( 'NONE', #11345, 1000.000000000000000 ) ;
#6506=CARTESIAN_POINT ( 'NONE',  ( -71.75000000204838102, 80.81189881250001861, -10.69163855873949132 ) ) ;
#6515=CARTESIAN_POINT ( 'NONE',  ( -73.34375000204839523, 55.00000000000000000, -25.81189881249999729 ) ) ;
#6516=CARTESIAN_POINT ( 'NONE',  ( -72.31250000409677625, 72.67766952966368876, 17.67766952966368521 ) ) ;
#6526=ORIENTED_EDGE ( 'NONE', *, *, #1881, .T. ) ;
#6535=ORIENTED_EDGE ( 'NONE', *, *, #7486, .T. ) ;
#6537=DIRECTION ( 'NONE',  ( -1.000000000000000000, 0.000000000000000000, -0.000000000000000000 ) ) ;
#6538=CIRCLE ( 'NONE', #8243, 27.53333900685068869 ) ;
#6542=CARTESIAN_POINT ( 'NONE',  ( -71.44842626887532333, 72.99142816090481745, 20.46173487478911568 ) ) ;
#6545=CARTESIAN_POINT ( 'NONE',  ( -76.25000000204838102, 65.69163855873948421, -25.81189881250000440 ) ) ;
#6552=EDGE_CURVE ( 'NONE', #10858, #8154, #6711, .T. ) ;
#6555=VECTOR ( 'NONE', #6962, 1000.000000000000000 ) ;
#6559=CARTESIAN_POINT ( 'NONE',  ( -71.99927362086853577, 76.65063509461015201, 12.50000000000143352 ) ) ;
#6565=CARTESIAN_POINT ( 'NONE',  ( -16.74007107453484622, 72.97142029985381839, -12.70283111168554235 ) ) ;
#6573=CARTESIAN_POINT ( 'NONE',  ( -76.43750000204839523, 44.30836144126050158, -25.81189881249999374 ) ) ;
#6577=ORIENTED_EDGE ( 'NONE', *, *, #8564, .T. ) ;
#6578=DIRECTION ( 'NONE',  ( 0.000000000000000000, 1.000000000000000000, 0.000000000000000000 ) ) ;
#6586=EDGE_CURVE ( 'NONE', #3987, #9278, #2921, .T. ) ;
#6602=DIRECTION ( 'NONE',  ( 0.000000000000000000, 0.000000000000000000, 1.000000000000000000 ) ) ;
#6603=CARTESIAN_POINT ( 'NONE',  ( -79.34375000204839523, 55.00000000000000000, -25.81189881249999729 ) ) ;
#6604=CARTESIAN_POINT ( 'NONE',  ( -72.40625000204838102, 29.18810118750000271, 4.741568889096522788E-15 ) ) ;
#6606=ORIENTED_EDGE ( 'NONE', *, *, #1024, .T. ) ;
#6607=CARTESIAN_POINT ( 'NONE',  ( -76.25000000409677625, 30.00000000000000355, 4.592425496802573578E-15 ) ) ;
#6609=CARTESIAN_POINT ( 'NONE',  ( 22.62790096952807772, 77.74555051095916269, -10.40404169996586958 ) ) ;
#6611=DIRECTION ( 'NONE',  ( 0.000000000000000000, 0.000000000000000000, -1.000000000000000000 ) ) ;
#6617=DIRECTION ( 'NONE',  ( -1.000000000000000000, -0.000000000000000000, -0.000000000000000000 ) ) ;
#6621=CARTESIAN_POINT ( 'NONE',  ( -5.009734977179735260, 65.88268349231633181, 19.12133901698799221 ) ) ;
#6623=EDGE_CURVE ( 'NONE', #9124, #10918, #6709, .T. ) ;
#6624=EDGE_LOOP ( 'NONE', ( #7634, #9749 ) ) ;
#6629=CARTESIAN_POINT ( 'NONE',  ( -78.78125000204839523, 73.25176868561975141, 18.25176868561974075 ) ) ;
#6633=LINE ( 'NONE', #381, #11587 ) ;
#6642=CARTESIAN_POINT ( 'NONE',  ( -76.06250000409679046, 37.32233047033631124, -17.67766952966368166 ) ) ;
#6652=CARTESIAN_POINT ( 'NONE',  ( -74.75000000409677625, 30.00000000000000355, 4.592425496802573578E-15 ) ) ;
#6660=CARTESIAN_POINT ( 'NONE',  ( -6.624926763187422019, 66.86059616939517980, 22.01099344385859879 ) ) ;
#6666=CARTESIAN_POINT ( 'NONE',  ( -76.90625000409677625, 80.00000000000001421, 10.35533905932737397 ) ) ;
#6668=CARTESIAN_POINT ( 'NONE',  ( 4.229223612318539161, 66.01664316016955070, -22.44374699675972451 ) ) ;
#6671=EDGE_CURVE ( 'NONE', #9881, #7673, #8772, .T. ) ;
#6677=CARTESIAN_POINT ( 'NONE',  ( -74.00000000000000000, 55.00000000000000000, -24.99999999999999645 ) ) ;
#6679=DIRECTION ( 'NONE',  ( 0.000000000000000000, 0.8660255361751957315, 0.4999997706924120267 ) ) ;
#6681=CARTESIAN_POINT ( 'NONE',  ( -73.06250000000008527, 37.32233047033641071, 17.67766952966358929 ) ) ;
#6684=ORIENTED_EDGE ( 'NONE', *, *, #542, .F. ) ;
#6687=ORIENTED_EDGE ( 'NONE', *, *, #3827, .F. ) ;
#6689=CARTESIAN_POINT ( 'NONE',  ( -75.96875000204839523, 80.81189881250000440, -1.580522963032174394E-15 ) ) ;
#6690=EDGE_CURVE ( 'NONE', #2686, #6077, #2142, .T. ) ;
#6693=CARTESIAN_POINT ( 'NONE',  ( -79.43750000000004263, 72.67766952966367455, 17.67766952966366745 ) ) ;
#6694=VECTOR ( 'NONE', #8438, 1000.000000000000000 ) ;
#6696=EDGE_LOOP ( 'NONE', ( #10050, #10340, #11791, #9995, #2567, #8898, #7779, #5843 ) ) ;
#6697=CARTESIAN_POINT ( 'NONE',  ( -73.53125000204839523, 36.74823131438024859, -18.25176868561973720 ) ) ;
#6698=ADVANCED_FACE ( 'NONE', ( #9260 ), #1052, .T. ) ;
#6699=PLANE ( 'NONE',  #8604 ) ;
#6707=AXIS2_PLACEMENT_3D ( 'NONE', #3362, #2184, #5854 ) ;
#6709=LINE ( 'NONE', #10339, #7891 ) ;
#6710=VERTEX_POINT ( 'NONE', #2478 ) ;
#6711=( BOUNDED_CURVE ( )  B_SPLINE_CURVE ( 2, ( #3754, #3817, #333, #3880, #4842, #272, #11108 ),
 .UNSPECIFIED., .F., .T. ) 
 B_SPLINE_CURVE_WITH_KNOTS ( ( 3, 2, 2, 3 ),
 ( 0.7921800998908017366, 0.8119924382482776037, 0.8318047766057536929, 0.8449751200525960071 ),
 .UNSPECIFIED. ) 
 CURVE ( )  GEOMETRIC_REPRESENTATION_ITEM ( )  RATIONAL_B_SPLINE_CURVE ( ( 1.000000000000000000, 0.9238795325112867385, 1.000000000000000000, 0.9238795325112867385, 1.000000000000000000, 0.9493985947158180005, 0.9660721892104719988 ) ) 
 REPRESENTATION_ITEM ( '' )  );
#6717=VERTEX_POINT ( 'NONE', #8834 ) ;
#6722=DIRECTION ( 'NONE',  ( 0.000000000000000000, 0.000000000000000000, -1.000000000000000000 ) ) ;
#6723=CARTESIAN_POINT ( 'NONE',  ( -20.92478415792846036, 76.34167033271135949, 13.02563361730251223 ) ) ;
#6725=CONICAL_SURFACE ( 'NONE', #8052, 17.04557674096337649, 0.1745329251994333364 ) ;
#6727=CARTESIAN_POINT ( 'NONE',  ( -73.06250000204840944, 80.81189881250001861, -10.69163855873949132 ) ) ;
#6729=CARTESIAN_POINT ( 'NONE',  ( 24.88384946230766559, 79.65201046289482179, -4.239228961464539758 ) ) ;
#6731=VECTOR ( 'NONE', #4154, 1000.000000000000000 ) ;
#6735=ORIENTED_EDGE ( 'NONE', *, *, #9371, .T. ) ;
#6738=CARTESIAN_POINT ( 'NONE',  ( -72.87500000000000000, 30.00000000000000355, 4.592425496802573578E-15 ) ) ;
#6750=CARTESIAN_POINT ( 'NONE',  ( -77.28125000204838102, 55.00000000000000000, 25.81189881249999729 ) ) ;
#6753=CARTESIAN_POINT ( 'NONE',  ( -75.50000000204840944, 44.30836144126053000, 25.81189881250000795 ) ) ;
#6757=CARTESIAN_POINT ( 'NONE',  ( -77.37500000409677625, 55.00000000000000000, -24.99999999999999645 ) ) ;
#6759=CARTESIAN_POINT ( 'NONE',  ( -73.06250000204842365, 80.81189881250000440, -10.69163855873948954 ) ) ;
#6761=DIRECTION ( 'NONE',  ( 0.000000000000000000, -0.000000000000000000, -1.000000000000000000 ) ) ;
#6780=CARTESIAN_POINT ( 'NONE',  ( -15.00000000000000000, -24.99999999999999645, -10.00000000000000000 ) ) ;
#6781=CARTESIAN_POINT ( 'NONE',  ( -78.96875000204839523, 80.81189881250000440, -1.580522963032174394E-15 ) ) ;
#6782=PLANE ( 'NONE',  #11449 ) ;
#6785=CARTESIAN_POINT ( 'NONE',  ( -73.53125000204839523, 36.74823131438024859, -18.25176868561973720 ) ) ;
#6789=EDGE_CURVE ( 'NONE', #4962, #10562, #6087, .T. ) ;
#6790=VECTOR ( 'NONE', #2621, 1000.000000000000000 ) ;
#6791=DIRECTION ( 'NONE',  ( 1.000000000000000000, 0.000000000000000000, 0.000000000000000000 ) ) ;
#6794=CARTESIAN_POINT ( 'NONE',  ( -73.62500000000000000, 80.00000000000000000, -1.530808498934191324E-15 ) ) ;
#6797=VERTEX_POINT ( 'NONE', #7936 ) ;
#6803=CARTESIAN_POINT ( 'NONE',  ( -78.21875000204839523, 36.74823131438024859, -18.25176868561973720 ) ) ;
#6806=CARTESIAN_POINT ( 'NONE',  ( -71.93750000204838102, 44.30836144126050158, -25.81189881249999374 ) ) ;
#6812=ORIENTED_EDGE ( 'NONE', *, *, #2586, .T. ) ;
#6814=EDGE_CURVE ( 'NONE', #6052, #388, #10731, .T. ) ;
#6816=DIRECTION ( 'NONE',  ( 0.000000000000000000, -1.000000000000000000, 0.000000000000000000 ) ) ;
#6822=CARTESIAN_POINT ( 'NONE',  ( -76.62500000409677625, 55.00000000000000000, 24.99999999999999645 ) ) ;
#6831=EDGE_CURVE ( 'NONE', #4892, #9278, #2597, .T. ) ;
#6836=DIRECTION ( 'NONE',  ( -1.000000000000000000, -0.000000000000000000, -0.000000000000000000 ) ) ;
#6838=CARTESIAN_POINT ( 'NONE',  ( -76.34375000204839523, 55.00000000000000000, -25.81189881249999729 ) ) ;
#6839=CARTESIAN_POINT ( 'NONE',  ( -75.87500000000007105, 30.00000000000010303, 4.592425496802555434E-15 ) ) ;
#6842=EDGE_CURVE ( 'NONE', #9989, #9742, #6265, .T. ) ;
#6844=CARTESIAN_POINT ( 'NONE',  ( -74.09375000204839523, 55.00000000000000000, 25.81189881249999729 ) ) ;
#6852=CARTESIAN_POINT ( 'NONE',  ( -73.25000000000000000, 55.00000000000000000, 24.99999999999999645 ) ) ;
#6853=ORIENTED_EDGE ( 'NONE', *, *, #8771, .F. ) ;
#6854=FACE_OUTER_BOUND ( 'NONE', #5100, .T. ) ;
#6855=CIRCLE ( 'NONE', #11224, 5.249999999999998224 ) ;
#6856=CARTESIAN_POINT ( 'NONE',  ( -73.25000000000000000, 55.00000000000000000, 24.99999999999999645 ) ) ;
#6863=CARTESIAN_POINT ( 'NONE',  ( 39.99999999999999289, 55.00000000000000000, -5.249999999999998224 ) ) ;
#6865=CARTESIAN_POINT ( 'NONE',  ( 0.7329934142408522924, 64.99605696851787684, 19.59792961213366169 ) ) ;
#6866=CARTESIAN_POINT ( 'NONE',  ( -79.06250000204839523, 80.81189881250000440, 10.69163855873948243 ) ) ;
#6867=ORIENTED_EDGE ( 'NONE', *, *, #64, .F. ) ;
#6868=CARTESIAN_POINT ( 'NONE',  ( -71.65625000204839523, 73.25176868561975141, -18.25176868561974430 ) ) ;
#6872=LINE ( 'NONE', #5734, #10250 ) ;
#6874=DIRECTION ( 'NONE',  ( -1.000000000000000000, -0.000000000000000000, -0.000000000000000000 ) ) ;
#6882=EDGE_LOOP ( 'NONE', ( #4471, #791 ) ) ;
#6889=VECTOR ( 'NONE', #8614, 1000.000000000000000 ) ;
#6894=CARTESIAN_POINT ( 'NONE',  ( -75.59375000204839523, 55.00000000000000000, 25.81189881249999729 ) ) ;
#6895=CARTESIAN_POINT ( 'NONE',  ( -12.39564893957180658, 69.98174787378947315, 20.04564381111873317 ) ) ;
#6898=CARTESIAN_POINT ( 'NONE',  ( -73.62500000409677625, 55.00000000000000000, 24.99999999999999645 ) ) ;
#6899=DIRECTION ( 'NONE',  ( 0.000000000000000000, 0.000000000000000000, -1.000000000000000000 ) ) ;
#6901=EDGE_LOOP ( 'NONE', ( #10421, #3838, #6914, #6853, #500, #1377 ) ) ;
#6910=CARTESIAN_POINT ( 'NONE',  ( -77.46875000000000000, 30.00000000000001421, 10.35533905932739174 ) ) ;
#6914=ORIENTED_EDGE ( 'NONE', *, *, #4700, .F. ) ;
#6917=AXIS2_PLACEMENT_3D ( 'NONE', #9218, #3834, #6602 ) ;
#6918=DIRECTION ( 'NONE',  ( 0.000000000000000000, 0.000000000000000000, 1.000000000000000000 ) ) ;
#6922=CARTESIAN_POINT ( 'NONE',  ( 4.665240958925800818, 65.77758632535075378, -19.17963262366009758 ) ) ;
#6924=CIRCLE ( 'NONE', #1739, 27.53333900685068869 ) ;
#6925=CARTESIAN_POINT ( 'NONE',  ( -77.00000000204839523, 29.18810118750000981, 10.69163855873950020 ) ) ;
#6929=CARTESIAN_POINT ( 'NONE',  ( -15.00000000000000000, 5.000000000000000000, -20.00000000000000000 ) ) ;
#6955=CARTESIAN_POINT ( 'NONE',  ( -76.43750000204839523, 44.30836144126049447, -25.81189881249999019 ) ) ;
#6960=CARTESIAN_POINT ( 'NONE',  ( -75.50000000409677625, 80.00000000000000000, -1.530808498934191324E-15 ) ) ;
#6961=CARTESIAN_POINT ( 'NONE',  ( 14.99999999999999645, 5.000000000000000000, 30.00000000000000711 ) ) ;
#6962=DIRECTION ( 'NONE',  ( -0.000000000000000000, -1.000000000000000000, -0.000000000000000000 ) ) ;
#6965=LINE ( 'NONE', #5887, #7228 ) ;
#6967=DIRECTION ( 'NONE',  ( 0.000000000000000000, 0.000000000000000000, -1.000000000000000000 ) ) ;
#6970=CARTESIAN_POINT ( 'NONE',  ( -73.53125000000000000, 80.00000000000001421, 10.35533905932737397 ) ) ;
#6973=DIRECTION ( 'NONE',  ( 0.000000000000000000, 0.000000000000000000, 1.000000000000000000 ) ) ;
#6978=ADVANCED_FACE ( 'NONE', ( #6380 ), #9177, .T. ) ;
#6980=CARTESIAN_POINT ( 'NONE',  ( 5.013139816730369347, 65.88383839924598817, 19.12068691178585311 ) ) ;
#6981=CARTESIAN_POINT ( 'NONE',  ( -77.75000000204839523, 80.81189881250000440, -10.69163855873948954 ) ) ;
#6982=ORIENTED_EDGE ( 'NONE', *, *, #111, .T. ) ;
#6989=EDGE_CURVE ( 'NONE', #10642, #11523, #9117, .T. ) ;
#6990=ORIENTED_EDGE ( 'NONE', *, *, #7785, .F. ) ;
#6996=CARTESIAN_POINT ( 'NONE',  ( -78.21875000204839523, 36.74823131438024859, -18.25176868561973720 ) ) ;
#7002=DIRECTION ( 'NONE',  ( 0.000000000000000000, 0.000000000000000000, -1.000000000000000000 ) ) ;
#7014=LINE ( 'NONE', #10637, #9958 ) ;
#7016=CARTESIAN_POINT ( 'NONE',  ( -72.03125000409679046, 44.64466094067237378, 24.99999999999975131 ) ) ;
#7021=CIRCLE ( 'NONE', #5293, 5.249999999999998224 ) ;
#7028=CARTESIAN_POINT ( 'NONE',  ( -77.75000000204839523, 80.81189881250001861, -10.69163855873949132 ) ) ;
#7041=CARTESIAN_POINT ( 'NONE',  ( 8.874488085748957644, 67.64441578773138986, -18.00748785805702212 ) ) ;
#7043=CARTESIAN_POINT ( 'NONE',  ( -75.12500000204838102, 44.30836144126049447, -25.81189881249999019 ) ) ;
#7051=AXIS2_PLACEMENT_3D ( 'NONE', #1973, #11129, #294 ) ;
#7053=ORIENTED_EDGE ( 'NONE', *, *, #5790, .F. ) ;
#7057=ORIENTED_EDGE ( 'NONE', *, *, #8583, .T. ) ;
#7060=CARTESIAN_POINT ( 'NONE',  ( -79.53125000204838102, 55.00000000000000000, -25.81189881249999729 ) ) ;
#7064=FILL_AREA_STYLE_COLOUR ( '', #7996 ) ;
#7069=ORIENTED_EDGE ( 'NONE', *, *, #4687, .T. ) ;
#7072=DIRECTION ( 'NONE',  ( 1.000000000000000000, 0.000000000000000000, 0.000000000000000000 ) ) ;
#7077=CARTESIAN_POINT ( 'NONE',  ( 14.99999999999999645, 0.000000000000000000, -10.00000000000000000 ) ) ;
#7082=EDGE_LOOP ( 'NONE', ( #2068, #3315, #7530, #4831, #6535, #4376, #2942, #7069, #2519, #8843, #4616, #5832 ) ) ;
#7085=DIRECTION ( 'NONE',  ( 1.000000000000000000, 0.000000000000000000, 0.000000000000000000 ) ) ;
#7090=CARTESIAN_POINT ( 'NONE',  ( -76.71875000204839523, 36.74823131438024859, -18.25176868561973720 ) ) ;
#7094=DIRECTION ( 'NONE',  ( 0.000000000000000000, 0.000000000000000000, -1.000000000000000000 ) ) ;
#7098=CARTESIAN_POINT ( 'NONE',  ( -15.00000000000000355, 5.000000000000000000, 20.00000000000000000 ) ) ;
#7099=VECTOR ( 'NONE', #10092, 1000.000000000000000 ) ;
#7101=CARTESIAN_POINT ( 'NONE',  ( -15.00000000000000000, -30.00000000000000000, 10.00000000000000000 ) ) ;
#7113=AXIS2_PLACEMENT_3D ( 'NONE', #4394, #4455, #11303 ) ;
#7118=CARTESIAN_POINT ( 'NONE',  ( -76.34375000204839523, 73.25176868561975141, -18.25176868561974430 ) ) ;
#7120=AXIS2_PLACEMENT_3D ( 'NONE', #6382, #6329, #11750 ) ;
#7124=( NAMED_UNIT ( * ) SI_UNIT ( $, .STERADIAN. ) SOLID_ANGLE_UNIT ( ) );
#7136=ORIENTED_EDGE ( 'NONE', *, *, #8112, .T. ) ;
#7137=CARTESIAN_POINT ( 'NONE',  ( -72.50000000409677625, 80.00000000000000000, -1.530808498934191324E-15 ) ) ;
#7143=ADVANCED_FACE ( 'NONE', ( #3129 ), #10370, .F. ) ;
#7144=CARTESIAN_POINT ( 'NONE',  ( -78.68750000409679046, 72.67766952966368876, -17.67766952966368876 ) ) ;
#7145=VERTEX_POINT ( 'NONE', #8588 ) ;
#7148=CARTESIAN_POINT ( 'NONE',  ( -71.99927368942448425, 76.65063862282433149, 12.49999388895319363 ) ) ;
#7150=ORIENTED_EDGE ( 'NONE', *, *, #668, .F. ) ;
#7153=CARTESIAN_POINT ( 'NONE',  ( 7.020400357098326438, 67.03996959729664695, 21.91068717264825239 ) ) ;
#7158=CARTESIAN_POINT ( 'NONE',  ( -75.21875000204839523, 36.74823131438024859, -18.25176868561973720 ) ) ;
#7169=AXIS2_PLACEMENT_3D ( 'NONE', #752, #10754, #3339 ) ;
#7171=ORIENTED_EDGE ( 'NONE', *, *, #668, .T. ) ;
#7173=CARTESIAN_POINT ( 'NONE',  ( -77.84375000204839523, 73.25176868561975141, -18.25176868561974430 ) ) ;
#7174=EDGE_LOOP ( 'NONE', ( #10747, #8294, #7859, #11142 ) ) ;
#7177=PRESENTATION_STYLE_ASSIGNMENT (( #2271 ) ) ;
#7186=DIRECTION ( 'NONE',  ( 0.000000000000000000, 0.000000000000000000, -1.000000000000000000 ) ) ;
#7190=CARTESIAN_POINT ( 'NONE',  ( -76.53125000000004263, 79.99999999999990052, 10.35533905932733312 ) ) ;
#7203=EDGE_CURVE ( 'NONE', #4769, #6710, #1206, .T. ) ;
#7206=CARTESIAN_POINT ( 'NONE',  ( -76.81250000204838102, 29.18810118750000626, -10.69163855873949309 ) ) ;
#7213=CARTESIAN_POINT ( 'NONE',  ( 1.722085729088277395, 65.52543047797470877, 22.67635561717434811 ) ) ;
#7218=CARTESIAN_POINT ( 'NONE',  ( -74.28125000204838102, 55.00000000000000000, 25.81189881249999729 ) ) ;
#7219=EDGE_LOOP ( 'NONE', ( #4877, #9251 ) ) ;
#7227=CARTESIAN_POINT ( 'NONE',  ( -15.35976620422333205, 71.92262103984167254, -14.06847932524695821 ) ) ;
#7228=VECTOR ( 'NONE', #8578, 1000.000000000000000 ) ;
#7233=VERTEX_POINT ( 'NONE', #305 ) ;
#7235=CARTESIAN_POINT ( 'NONE',  ( -74.46875000204839523, 73.25176868561975141, 18.25176868561974075 ) ) ;
#7241=ADVANCED_FACE ( 'NONE', ( #3537 ), #8820, .F. ) ;
#7256=ORIENTED_EDGE ( 'NONE', *, *, #2521, .T. ) ;
#7259=CARTESIAN_POINT ( 'NONE',  ( 36.99999999999999289, 55.00000000000000000, -5.249999999999998224 ) ) ;
#7262=CARTESIAN_POINT ( 'NONE',  ( -75.03125000204838102, 55.00000000000000000, -25.81189881249999729 ) ) ;
#7265=CARTESIAN_POINT ( 'NONE',  ( -74.65625000204839523, 73.25176868561975141, -18.25176868561974430 ) ) ;
#7267=CARTESIAN_POINT ( 'NONE',  ( 21.38655605994216558, 76.71840771742046172, 12.40410437900267127 ) ) ;
#7272=CARTESIAN_POINT ( 'NONE',  ( 6.123233995736766282E-16, -30.00000000000000000, 5.000000000000000000 ) ) ;
#7283=CARTESIAN_POINT ( 'NONE',  ( -21.12429042622422060, 76.50559246739102548, 4.651484971764126009 ) ) ;
#7290=CARTESIAN_POINT ( 'NONE',  ( -76.15625000204839523, 73.25176868561975141, -18.25176868561974430 ) ) ;
#7315=CARTESIAN_POINT ( 'NONE',  ( -74.46875000409679046, 44.64466094067277879, -25.00000000000015987 ) ) ;
#7320=CARTESIAN_POINT ( 'NONE',  ( -73.53125000204838102, 55.00000000000000000, -25.81189881249999729 ) ) ;
#7325=VERTEX_POINT ( 'NONE', #5344 ) ;
#7330=CARTESIAN_POINT ( 'NONE',  ( -78.96875000000001421, 30.00000000000003908, 10.35533905932737753 ) ) ;
#7339=PLANE ( 'NONE',  #7120 ) ;
#7342=ORIENTED_EDGE ( 'NONE', *, *, #542, .T. ) ;
#7346=CARTESIAN_POINT ( 'NONE',  ( -78.50000000204840944, 44.30836144126053000, 25.81189881250000795 ) ) ;
#7363=DIRECTION ( 'NONE',  ( -1.000000000000000000, -0.000000000000000000, -0.000000000000000000 ) ) ;
#7372=CARTESIAN_POINT ( 'NONE',  ( -73.25000000204838102, 80.81189881250001861, -10.69163855873949132 ) ) ;
#7376=CARTESIAN_POINT ( 'NONE',  ( -75.59375000204839523, 55.00000000000000000, 25.81189881249999729 ) ) ;
#7378=CARTESIAN_POINT ( 'NONE',  ( 5.849089671321329398, 66.56396111897267076, 22.16541920639843255 ) ) ;
#7381=CARTESIAN_POINT ( 'NONE',  ( 39.99999999999999289, 55.00000000000000000, 0.000000000000000000 ) ) ;
#7386=CARTESIAN_POINT ( 'NONE',  ( -74.09375000000007105, 44.64466094067265800, -24.99999999999985434 ) ) ;
#7391=CARTESIAN_POINT ( 'NONE',  ( -18.38663302488769347, 74.26727426732456649, 10.62400905199263690 ) ) ;
#7396=DIRECTION ( 'NONE',  ( -0.000000000000000000, -1.000000000000000000, -0.000000000000000000 ) ) ;
#7398=CARTESIAN_POINT ( 'NONE',  ( -74.00000000409677625, 80.00000000000000000, -1.530808498934191324E-15 ) ) ;
#7401=CARTESIAN_POINT ( 'NONE',  ( -72.31250000204839523, 29.18810118750000626, -10.69163855873949309 ) ) ;
#7402=VERTEX_POINT ( 'NONE', #8936 ) ;
#7410=EDGE_CURVE ( 'NONE', #4040, #5487, #11685, .T. ) ;
#7411=CARTESIAN_POINT ( 'NONE',  ( -72.50000000409677625, 80.00000000000000000, -1.530808498934191324E-15 ) ) ;
#7413=ORIENTED_EDGE ( 'NONE', *, *, #11763, .F. ) ;
#7417=CARTESIAN_POINT ( 'NONE',  ( -73.15625000409679046, 30.00000000000000355, -10.35533905932738108 ) ) ;
#7422=CARTESIAN_POINT ( 'NONE',  ( 36.99999999999999289, 55.00000000000000000, 0.000000000000000000 ) ) ;
#7425=CARTESIAN_POINT ( 'NONE',  ( -71.18750000409677625, 72.67766952966368876, -17.67766952966368876 ) ) ;
#7432=ORIENTED_EDGE ( 'NONE', *, *, #7701, .T. ) ;
#7437=CARTESIAN_POINT ( 'NONE',  ( -0.4307873465902548049, 65.42943686846950868, -22.72062601704910989 ) ) ;
#7441=CARTESIAN_POINT ( 'NONE',  ( -79.06250000204840944, 80.81189881250001861, -10.69163855873949132 ) ) ;
#7443=CARTESIAN_POINT ( 'NONE',  ( 8.136848973421107800, 67.55742525566687107, -21.61847732402205580 ) ) ;
#7447=EDGE_CURVE ( 'NONE', #10129, #11498, #1552, .T. ) ;
#7449=LINE ( 'NONE', #2036, #1496 ) ;
#7451=CARTESIAN_POINT ( 'NONE',  ( -79.81250000000001421, 72.67766952966368876, -17.67766952966368876 ) ) ;
#7458=CARTESIAN_POINT ( 'NONE',  ( -20.36561017906013404, 75.87354305742351812, -7.076759675131881977 ) ) ;
#7468=CARTESIAN_POINT ( 'NONE',  ( -76.81250000204839523, 29.18810118750000981, 10.69163855873950020 ) ) ;
#7469=ADVANCED_FACE ( 'NONE', ( #1971 ), #10803, .F. ) ;
#7478=DIRECTION ( 'NONE',  ( 1.000000000000000000, 0.000000000000000000, 0.000000000000000000 ) ) ;
#7486=EDGE_CURVE ( 'NONE', #4282, #9278, #7014, .T. ) ;
#7491=CARTESIAN_POINT ( 'NONE',  ( -77.37500000000005684, 30.00000000000009592, 4.592425496802557801E-15 ) ) ;
#7492=AXIS2_PLACEMENT_3D ( 'NONE', #9445, #7544, #153 ) ;
#7500=CARTESIAN_POINT ( 'NONE',  ( -14.95549379722967487, 71.72953881524270514, -18.61174932058436582 ) ) ;
#7502=VERTEX_POINT ( 'NONE', #7077 ) ;
#7503=CARTESIAN_POINT ( 'NONE',  ( -76.15625000409677625, 30.00000000000000355, -10.35533905932738108 ) ) ;
#7504=VECTOR ( 'NONE', #2841, 1000.000000000000000 ) ;
#7506=CARTESIAN_POINT ( 'NONE',  ( 25.02328063624275600, 79.77146175834676001, 3.399146611245127847 ) ) ;
#7514=CARTESIAN_POINT ( 'NONE',  ( -78.78125000000001421, 30.00000000000000355, -10.35533905932738108 ) ) ;
#7526=CARTESIAN_POINT ( 'NONE',  ( -78.96875000204839523, 80.81189881250000440, -1.580522963032174394E-15 ) ) ;
#7527=DIRECTION ( 'NONE',  ( 0.000000000000000000, 0.000000000000000000, 1.000000000000000000 ) ) ;
#7530=ORIENTED_EDGE ( 'NONE', *, *, #6789, .F. ) ;
#7531=CARTESIAN_POINT ( 'NONE',  ( -74.09375000204839523, 55.00000000000000000, 25.81189881249999729 ) ) ;
#7535=ORIENTED_EDGE ( 'NONE', *, *, #7203, .T. ) ;
#7543=ORIENTED_EDGE ( 'NONE', *, *, #6690, .T. ) ;
#7544=DIRECTION ( 'NONE',  ( 0.000000000000000000, 1.000000000000000000, 0.000000000000000000 ) ) ;
#7553=CARTESIAN_POINT ( 'NONE',  ( -15.00000000000000000, 55.00000000000000000, 0.000000000000000000 ) ) ;
#7556=CARTESIAN_POINT ( 'NONE',  ( -8.153690333911775667, 67.55523279586272167, -21.62223061169231997 ) ) ;
#7560=CARTESIAN_POINT ( 'NONE',  ( -78.31250000409679046, 72.67766952966368876, 17.67766952966368521 ) ) ;
#7562=CARTESIAN_POINT ( 'NONE',  ( 9.245291525937640031, 68.12702208362456702, -21.27760407867818770 ) ) ;
#7564=CARTESIAN_POINT ( 'NONE',  ( 14.99999999999999645, 0.000000000000000000, 30.00000000000000711 ) ) ;
#7566=EDGE_CURVE ( 'NONE', #7233, #9881, #2635, .T. ) ;
#7567=EDGE_CURVE ( 'NONE', #8679, #9967, #8761, .T. ) ;
#7573=LINE ( 'NONE', #6961, #1521 ) ;
#7577=CARTESIAN_POINT ( 'NONE',  ( -73.25000000000000000, 55.00000000000000000, 24.99999999999999645 ) ) ;
#7579=ORIENTED_EDGE ( 'NONE', *, *, #9671, .F. ) ;
#7584=CARTESIAN_POINT ( 'NONE',  ( -75.40625000204839523, 36.74823131438026280, 18.25176868561974786 ) ) ;
#7586=CARTESIAN_POINT ( 'NONE',  ( -80.00000000000000000, 55.00000000000000000, -24.99999999999999645 ) ) ;
#7613=CARTESIAN_POINT ( 'NONE',  ( -24.87631665557734095, 79.64556585907233455, -4.276919348231523976 ) ) ;
#7616=AXIS2_PLACEMENT_3D ( 'NONE', #372, #4037, #3914 ) ;
#7617=CARTESIAN_POINT ( 'NONE',  ( -71.75000000204840944, 65.69163855873948421, -25.81189881250000440 ) ) ;
#7619=CARTESIAN_POINT ( 'NONE',  ( 24.23505289248274863, 79.09914288581300923, -6.663429661133934978 ) ) ;
#7625=EDGE_LOOP ( 'NONE', ( #6154, #10894, #5544, #7342, #526 ) ) ;
#7626=CARTESIAN_POINT ( 'NONE',  ( -77.56250000000000000, 37.32233047033631124, 17.67766952966369232 ) ) ;
#7632=CARTESIAN_POINT ( 'NONE',  ( -12.32394926038158012, 69.76387561330639642, 16.31736050817429984 ) ) ;
#7634=ORIENTED_EDGE ( 'NONE', *, *, #1959, .T. ) ;
#7636=CARTESIAN_POINT ( 'NONE',  ( -78.03125000204838102, 55.00000000000000000, -25.81189881249999729 ) ) ;
#7641=CARTESIAN_POINT ( 'NONE',  ( -73.43750000204839523, 44.30836144126050158, -25.81189881249999374 ) ) ;
#7646=CARTESIAN_POINT ( 'NONE',  ( -77.46875000409679046, 44.64466094067266511, -25.00000000000004263 ) ) ;
#7648=DIRECTION ( 'NONE',  ( 0.000000000000000000, 0.000000000000000000, 1.000000000000000000 ) ) ;
#7658=ORIENTED_EDGE ( 'NONE', *, *, #8437, .F. ) ;
#7664=CARTESIAN_POINT ( 'NONE',  ( 39.99999999999999289, 55.00000000000000000, 0.000000000000000000 ) ) ;
#7666=EDGE_LOOP ( 'NONE', ( #2979, #11069, #2949, #6352 ) ) ;
#7670=CARTESIAN_POINT ( 'NONE',  ( -75.21875000204839523, 29.18810118750000271, 4.741568889096522788E-15 ) ) ;
#7673=VERTEX_POINT ( 'NONE', #31 ) ;
#7674=CARTESIAN_POINT ( 'NONE',  ( -77.28125000409677625, 65.35533905932737753, -24.99999999999999645 ) ) ;
#7676=CARTESIAN_POINT ( 'NONE',  ( 16.74161068948953357, 73.05576634196897601, -17.30319104633145955 ) ) ;
#7684=CARTESIAN_POINT ( 'NONE',  ( -74.18750000000000000, 37.32233047033631124, -17.67766952966368166 ) ) ;
#7696=CARTESIAN_POINT ( 'NONE',  ( -78.59375000204839523, 36.74823131438026280, 18.25176868561974786 ) ) ;
#7699=CARTESIAN_POINT ( 'NONE',  ( -71.40810441781462714, 80.81189881250000440, 6.916273779317701376 ) ) ;
#7701=EDGE_CURVE ( 'NONE', #10478, #884, #4656, .T. ) ;
#7702=EDGE_CURVE ( 'NONE', #8432, #3359, #5971, .T. ) ;
#7703=CARTESIAN_POINT ( 'NONE',  ( -75.68750000409677625, 72.67766952966368876, -17.67766952966368876 ) ) ;
#7710=ADVANCED_FACE ( 'NONE', ( #8309, #1055 ), #2194, .F. ) ;
#7721=ORIENTED_EDGE ( 'NONE', *, *, #10757, .F. ) ;
#7729=CARTESIAN_POINT ( 'NONE',  ( 14.99999999999999645, 0.000000000000000000, 30.00000000000000711 ) ) ;
#7730=CARTESIAN_POINT ( 'NONE',  ( -74.93750000204838102, 44.30836144126049447, -25.81189881249999019 ) ) ;
#7731=CARTESIAN_POINT ( 'NONE',  ( -24.88738022673829775, 79.65503066217630135, 4.221719104015677182 ) ) ;
#7734=CARTESIAN_POINT ( 'NONE',  ( -76.62500000409677625, 55.00000000000000000, 24.99999999999999645 ) ) ;
#7741=CARTESIAN_POINT ( 'NONE',  ( -73.53125000000005684, 79.99999999999987210, 10.35533905932731891 ) ) ;
#7743=CARTESIAN_POINT ( 'NONE',  ( -76.53124999999998579, 80.00000000000001421, 10.35533905932737397 ) ) ;
#7746=ORIENTED_EDGE ( 'NONE', *, *, #140, .T. ) ;
#7748=CARTESIAN_POINT ( 'NONE',  ( -3.970850827666276395, 65.56567621485199027, 19.29717822822915707 ) ) ;
#7750=CARTESIAN_POINT ( 'NONE',  ( 7.008258234807173359, 66.69771099951718440, 18.63519012541959441 ) ) ;
#7752=ORIENTED_EDGE ( 'NONE', *, *, #3418, .T. ) ;
#7769=AXIS2_PLACEMENT_3D ( 'NONE', #3890, #11175, #5874 ) ;
#7777=FACE_OUTER_BOUND ( 'NONE', #2234, .T. ) ;
#7779=ORIENTED_EDGE ( 'NONE', *, *, #2839, .F. ) ;
#7785=EDGE_CURVE ( 'NONE', #6797, #30, #4828, .T. ) ;
#7786=CARTESIAN_POINT ( 'NONE',  ( -76.06250000204842365, 80.81189881250000440, -10.69163855873948954 ) ) ;
#7787=CARTESIAN_POINT ( 'NONE',  ( -20.69108674001310177, 76.15158908439804009, 13.33178032960098314 ) ) ;
#7798=VERTEX_POINT ( 'NONE', #135 ) ;
#7799=CARTESIAN_POINT ( 'NONE',  ( 14.99999999999999645, 5.000000000000000000, -29.99999999999999289 ) ) ;
#7801=CARTESIAN_POINT ( 'NONE',  ( -75.68750000000000000, 37.32233047033631124, -17.67766952966368166 ) ) ;
#7805=EDGE_CURVE ( 'NONE', #2575, #4892, #9307, .T. ) ;
#7810=ORIENTED_EDGE ( 'NONE', *, *, #4675, .F. ) ;
#7811=CARTESIAN_POINT ( 'NONE',  ( 21.36911699583331270, 76.71007065292897664, -3.630805090811919378 ) ) ;
#7813=VERTEX_POINT ( 'NONE', #9427 ) ;
#7814=CARTESIAN_POINT ( 'NONE',  ( -76.06250000204840944, 80.81189881250001861, -10.69163855873949132 ) ) ;
#7845=CARTESIAN_POINT ( 'NONE',  ( 9.999999999999994671, 0.000000000000000000, -10.00000000000000000 ) ) ;
#7846=CARTESIAN_POINT ( 'NONE',  ( -74.84375000204839523, 55.00000000000000000, -25.81189881249999729 ) ) ;
#7847=CARTESIAN_POINT ( 'NONE',  ( -16.74856700446162705, 73.06100190697902974, 17.29768990044683363 ) ) ;
#7850=CARTESIAN_POINT ( 'NONE',  ( -72.59375000409677625, 80.00000000000001421, -10.35533905932737753 ) ) ;
#7853=VECTOR ( 'NONE', #11460, 1000.000000000000000 ) ;
#7855=CARTESIAN_POINT ( 'NONE',  ( -75.03125000000005684, 79.99999999999990052, 10.35533905932732779 ) ) ;
#7856=DIRECTION ( 'NONE',  ( 0.000000000000000000, 0.000000000000000000, -1.000000000000000000 ) ) ;
#7859=ORIENTED_EDGE ( 'NONE', *, *, #7702, .T. ) ;
#7861=CARTESIAN_POINT ( 'NONE',  ( -74.93750000000000000, 72.67766952966368876, 17.67766952966368521 ) ) ;
#7876=CARTESIAN_POINT ( 'NONE',  ( -77.56250000204838102, 80.81189881250000440, 10.69163855873948243 ) ) ;
#7880=CARTESIAN_POINT ( 'NONE',  ( -75.78125000409680467, 65.35533905932749121, -24.99999999999989342 ) ) ;
#7891=VECTOR ( 'NONE', #2978, 1000.000000000000000 ) ;
#7892=CARTESIAN_POINT ( 'NONE',  ( -74.56250000204839523, 80.81189881250001861, 10.69163855873948599 ) ) ;
#7896=ADVANCED_FACE ( 'NONE', ( #2178 ), #10324, .T. ) ;
#7897=DIRECTION ( 'NONE',  ( 1.000000000000000000, -0.000000000000000000, 0.000000000000000000 ) ) ;
#7906=CARTESIAN_POINT ( 'NONE',  ( -76.62500000204838102, 29.18810118750000626, -10.69163855873949132 ) ) ;
#7910=CARTESIAN_POINT ( 'NONE',  ( -75.78125000409680467, 65.35533905932737753, -24.99999999999999645 ) ) ;
#7917=CARTESIAN_POINT ( 'NONE',  ( -15.00000000000000000, -30.00000000000000000, 10.00000000000000000 ) ) ;
#7920=CARTESIAN_POINT ( 'NONE',  ( -77.28125000204838102, 55.00000000000000000, 25.81189881249999729 ) ) ;
#7921=DIRECTION ( 'NONE',  ( -0.000000000000000000, -1.000000000000000000, -0.000000000000000000 ) ) ;
#7922=ORIENTED_EDGE ( 'NONE', *, *, #1959, .F. ) ;
#7925=( BOUNDED_CURVE ( )  B_SPLINE_CURVE ( 2, ( #1463, #7880, #7703, #8713, #5125, #552, #5907, #9550, #4218 ),
 .UNSPECIFIED., .F., .T. ) 
 B_SPLINE_CURVE_WITH_KNOTS ( ( 3, 2, 2, 2, 3 ),
 ( 0.3333333333333335924, 0.3541666666666669627, 0.3750000000000003331, 0.3958333333333336479, 0.4166666666666670182 ),
 .UNSPECIFIED. ) 
 CURVE ( )  GEOMETRIC_REPRESENTATION_ITEM ( )  RATIONAL_B_SPLINE_CURVE ( ( 0.9999999999999990008, 0.9238795325112877377, 1.000000000000000000, 0.9238795325112867385, 1.000000000000000000, 0.9238795325112867385, 1.000000000000000000, 0.9238795325112855172, 1.000000000000001110 ) ) 
 REPRESENTATION_ITEM ( '' )  );
#7931=CARTESIAN_POINT ( 'NONE',  ( 13.89805254290603109, 70.85503171694512048, 15.26047230127977627 ) ) ;
#7932=CARTESIAN_POINT ( 'NONE',  ( -74.56250000204839523, 80.81189881250000440, 10.69163855873948243 ) ) ;
#7936=CARTESIAN_POINT ( 'NONE',  ( -77.75000000000000000, 55.00000000000000000, 24.99999999999999645 ) ) ;
#7943=( BOUNDED_CURVE ( )  B_SPLINE_CURVE ( 2, ( #1558, #5048, #5105, #419, #1387, #7741, #3297, #3125, #6852 ),
 .UNSPECIFIED., .F., .T. ) 
 B_SPLINE_CURVE_WITH_KNOTS ( ( 3, 2, 2, 2, 3 ),
 ( 0.6337432032608648624, 0.6535433226934000972, 0.6733434421259354430, 0.6931435615584705667, 0.7129436809910058015 ),
 .UNSPECIFIED. ) 
 CURVE ( )  GEOMETRIC_REPRESENTATION_ITEM ( )  RATIONAL_B_SPLINE_CURVE ( ( 1.000000000000000000, 0.9238795325112868495, 1.000000000000000000, 0.9238795325112868495, 1.000000000000000000, 0.9238795325112868495, 1.000000000000000000, 0.9238795325112868495, 1.000000000000000000 ) ) 
 REPRESENTATION_ITEM ( '' )  );
#7944=ORIENTED_EDGE ( 'NONE', *, *, #4324, .F. ) ;
#7947=CARTESIAN_POINT ( 'NONE',  ( -78.03125000204838102, 55.00000000000000000, -25.81189881249999729 ) ) ;
#7959=CARTESIAN_POINT ( 'NONE',  ( -80.00000000000000000, 55.00000000000000000, 0.000000000000000000 ) ) ;
#7960=CARTESIAN_POINT ( 'NONE',  ( 0.000000000000000000, 50.00000000000000000, 0.000000000000000000 ) ) ;
#7962=VERTEX_POINT ( 'NONE', #3372 ) ;
#7963=CARTESIAN_POINT ( 'NONE',  ( -73.06250000409677625, 37.32233047033631124, -17.67766952966368166 ) ) ;
#7976=CARTESIAN_POINT ( 'NONE',  ( -79.15625000204838102, 80.81189881250000440, -1.580522963032174394E-15 ) ) ;
#7979=AXIS2_PLACEMENT_3D ( 'NONE', #3003, #11009, #112 ) ;
#7985=CARTESIAN_POINT ( 'NONE',  ( 5.696514063848578502, 66.13915503709409904, 18.97435054747177574 ) ) ;
#7986=CARTESIAN_POINT ( 'NONE',  ( -71.53052369147287948, 77.35376373433385311, 12.90594309674112772 ) ) ;
#7990=( BOUNDED_CURVE ( )  B_SPLINE_CURVE ( 2, ( #5103, #1438, #8692, #474, #8749, #7855, #937, #2632, #10882 ),
 .UNSPECIFIED., .F., .T. ) 
 B_SPLINE_CURVE_WITH_KNOTS ( ( 3, 2, 2, 2, 3 ),
 ( 0.4753074076738947884, 0.4951072852372784272, 0.5149071628006619550, 0.5347070403640455938, 0.5545069179274292326 ),
 .UNSPECIFIED. ) 
 CURVE ( )  GEOMETRIC_REPRESENTATION_ITEM ( )  RATIONAL_B_SPLINE_CURVE ( ( 1.000000000000002220, 0.9238795325112845180, 1.000000000000000000, 0.9238795325112867385, 1.000000000000000000, 0.9238795325112867385, 1.000000000000000000, 0.9238795325113021706, 0.9999999999999845679 ) ) 
 REPRESENTATION_ITEM ( '' )  );
#7991=CARTESIAN_POINT ( 'NONE',  ( 39.99999999999999289, 55.00000000000000000, 24.99999999999999645 ) ) ;
#7996=COLOUR_RGB ( '',0.8941176470588234615, 0.8941176470588234615, 0.8941176470588234615 ) ;
#8000=EDGE_CURVE ( 'NONE', #3514, #11523, #6088, .T. ) ;
#8005=CARTESIAN_POINT ( 'NONE',  ( -76.53125000204838102, 55.00000000000000000, -25.81189881249999729 ) ) ;
#8011=DIRECTION ( 'NONE',  ( 0.000000000000000000, 0.000000000000000000, 1.000000000000000000 ) ) ;
#8017=DIRECTION ( 'NONE',  ( 0.000000000000000000, -0.000000000000000000, -1.000000000000000000 ) ) ;
#8023=CARTESIAN_POINT ( 'NONE',  ( -74.84375000409679046, 30.00000000000001421, 10.35533905932739174 ) ) ;
#8035=CARTESIAN_POINT ( 'NONE',  ( -74.75000000204839523, 80.81189881250001861, -10.69163855873949132 ) ) ;
#8038=VERTEX_POINT ( 'NONE', #11333 ) ;
#8043=CARTESIAN_POINT ( 'NONE',  ( -80.00000000000000000, 55.00000000000000000, -22.00000000000000000 ) ) ;
#8046=CARTESIAN_POINT ( 'NONE',  ( -75.03125000204838102, 55.00000000000000000, -25.81189881249999729 ) ) ;
#8052=AXIS2_PLACEMENT_3D ( 'NONE', #10210, #3927, #3873 ) ;
#8064=CARTESIAN_POINT ( 'NONE',  ( -75.96875000204839523, 73.25176868561975141, 18.25176868561974075 ) ) ;
#8084=CARTESIAN_POINT ( 'NONE',  ( 0.000000000000000000, 50.00000000000000000, 20.00000000000000000 ) ) ;
#8085=DIRECTION ( 'NONE',  ( -1.000000000000000000, -0.000000000000000000, -0.000000000000000000 ) ) ;
#8094=PLANE ( 'NONE',  #10061 ) ;
#8098=CARTESIAN_POINT ( 'NONE',  ( -76.43750000204838102, 65.69163855873948421, -25.81189881250000440 ) ) ;
#8101=DIRECTION ( 'NONE',  ( 1.000000000000000000, 0.000000000000000000, 0.000000000000000000 ) ) ;
#8105=DIRECTION ( 'NONE',  ( 0.000000000000000000, 0.000000000000000000, -1.000000000000000000 ) ) ;
#8108=CARTESIAN_POINT ( 'NONE',  ( -74.46875000204839523, 73.25176868561975141, 18.25176868561974075 ) ) ;
#8112=EDGE_CURVE ( 'NONE', #884, #9742, #7925, .T. ) ;
#8115=CARTESIAN_POINT ( 'NONE',  ( -9.472297265023270185, 67.98144036619800090, -17.76723545671738336 ) ) ;
#8122=CARTESIAN_POINT ( 'NONE',  ( -74.75000000204839523, 80.81189881250001861, -10.69163855873949132 ) ) ;
#8132=DIRECTION ( 'NONE',  ( 1.000000000000000000, 0.000000000000000000, 0.000000000000000000 ) ) ;
#8138=DIRECTION ( 'NONE',  ( 0.000000000000000000, -1.000000000000000000, 0.000000000000000000 ) ) ;
#8141=ORIENTED_EDGE ( 'NONE', *, *, #7567, .F. ) ;
#8149=CARTESIAN_POINT ( 'NONE',  ( -78.40625000204838102, 29.18810118750000271, 4.741568889096522788E-15 ) ) ;
#8153=CARTESIAN_POINT ( 'NONE',  ( -79.34375000204839523, 55.00000000000000000, -25.81189881249999729 ) ) ;
#8154=VERTEX_POINT ( 'NONE', #10732 ) ;
#8155=CARTESIAN_POINT ( 'NONE',  ( 19.48027454407776915, 75.17671222592493052, 14.77705221063085617 ) ) ;
#8158=CARTESIAN_POINT ( 'NONE',  ( -77.18750000409679046, 72.67766952966368876, -17.67766952966368876 ) ) ;
#8161=ORIENTED_EDGE ( 'NONE', *, *, #996, .T. ) ;
#8170=CARTESIAN_POINT ( 'NONE',  ( -0.7352373834349590354, 64.99605696851786263, -19.59792961213366169 ) ) ;
#8174=EDGE_LOOP ( 'NONE', ( #2074, #6606, #4562, #2278 ) ) ;
#8175=CARTESIAN_POINT ( 'NONE',  ( 9.999999999999994671, -30.00000000000000000, 10.00000000000000000 ) ) ;
#8178=CARTESIAN_POINT ( 'NONE',  ( -72.21875000204838102, 36.74823131438024859, -18.25176868561973720 ) ) ;
#8180=CIRCLE ( 'NONE', #10653, 5.000000000000000000 ) ;
#8185=ORIENTED_EDGE ( 'NONE', *, *, #9896, .F. ) ;
#8198=CARTESIAN_POINT ( 'NONE',  ( -71.00000000409677625, 80.00000000000000000, -1.530808498934191324E-15 ) ) ;
#8207=CARTESIAN_POINT ( 'NONE',  ( -71.65625000204838102, 80.81189881250000440, -1.580522963032174394E-15 ) ) ;
#8211=EDGE_CURVE ( 'NONE', #7233, #9521, #2540, .T. ) ;
#8212=CARTESIAN_POINT ( 'NONE',  ( -74.75000000204840944, 65.69163855873948421, -25.81189881250000440 ) ) ;
#8213=EDGE_LOOP ( 'NONE', ( #1458, #1433, #6812, #9504 ) ) ;
#8218=CARTESIAN_POINT ( 'NONE',  ( -76.90625000409677625, 80.00000000000001421, 10.35533905932737397 ) ) ;
#8224=CARTESIAN_POINT ( 'NONE',  ( -71.53052369147287948, 77.35376373433385311, 12.90594309674112772 ) ) ;
#8229=AXIS2_PLACEMENT_3D ( 'NONE', #4263, #7921, #1503 ) ;
#8230=CARTESIAN_POINT ( 'NONE',  ( -18.91777915131708454, 74.69377696386850118, -9.811015657242856847 ) ) ;
#8237=CARTESIAN_POINT ( 'NONE',  ( -78.59375000204839523, 55.00000000000000000, 25.81189881249999729 ) ) ;
#8243=AXIS2_PLACEMENT_3D ( 'NONE', #3833, #343, #9334 ) ;
#8255=CARTESIAN_POINT ( 'NONE',  ( -71.28125000409676204, 65.35533905932761911, -24.99999999999974420 ) ) ;
#8267=CARTESIAN_POINT ( 'NONE',  ( -3.411829342377862062, 65.82156647569453867, -22.53680681160409094 ) ) ;
#8270=CARTESIAN_POINT ( 'NONE',  ( -77.18750000204839523, 65.69163855873949842, 25.81189881250000440 ) ) ;
#8275=LINE ( 'NONE', #11133, #11215 ) ;
#8278=CARTESIAN_POINT ( 'NONE',  ( -79.34375000000002842, 65.35533905932737753, 24.99999999999999645 ) ) ;
#8284=CARTESIAN_POINT ( 'NONE',  ( -8.864316419551519388, 67.63873506485967368, -18.01151076427558806 ) ) ;
#8293=CARTESIAN_POINT ( 'NONE',  ( -77.56250000204839523, 80.81189881250001861, -10.69163855873949132 ) ) ;
#8294=ORIENTED_EDGE ( 'NONE', *, *, #10321, .T. ) ;
#8305=DIRECTION ( 'NONE',  ( 0.000000000000000000, 0.9848077530122080203, 0.1736481776669307198 ) ) ;
#8307=CYLINDRICAL_SURFACE ( 'NONE', #11077, 5.000000000000000000 ) ;
#8309=FACE_BOUND ( 'NONE', #9058, .T. ) ;
#8313=CARTESIAN_POINT ( 'NONE',  ( -74.84375000409676204, 30.00000000000001421, 10.35533905932739174 ) ) ;
#8317=CARTESIAN_POINT ( 'NONE',  ( -72.03125000204838102, 55.00000000000000000, -25.81189881249999729 ) ) ;
#8320=CARTESIAN_POINT ( 'NONE',  ( -72.87500000204839523, 65.69163855873949842, 25.81189881250000440 ) ) ;
#8324=CARTESIAN_POINT ( 'NONE',  ( -77.93750000204838102, 44.30836144126050158, -25.81189881249999374 ) ) ;
#8325=ORIENTED_EDGE ( 'NONE', *, *, #2866, .F. ) ;
#8326=CARTESIAN_POINT ( 'NONE',  ( 11.04711134339418876, 69.12045815601207721, -20.65175458094307004 ) ) ;
#8339=CARTESIAN_POINT ( 'NONE',  ( -17.99829699906814184, 73.95811728008973773, 11.16634296551433714 ) ) ;
#8349=CARTESIAN_POINT ( 'NONE',  ( -77.09375000204839523, 55.00000000000000000, 25.81189881249999729 ) ) ;
#8354=B_SPLINE_CURVE_WITH_KNOTS ( 'NONE', 3,
 ( #3769, #7437, #4794, #11064, #5454, #10231, #8267, #10947, #2757, #3894, #10999, #7556, #6416, #1845, #9273, #165, #2875, #7500, #2935, #2025, #5513, #11179, #11124, #5699, #9160, #9337, #2811, #10106, #1906, #5574, #11475, #1310, #8741, #7613, #5761, #4124, #9398, #5822, #9459, #11242, #4074, #3053, #7731, #3951, #4976, #10293, #9579, #1193, #4857, #5094, #5038, #6723, #7787, #8685, #9635, #7847, #10523, #10354, #2151, #6895, #467, #1375, #11416, #6660, #3227, #1431, #2331, #346, #1245, #524, #6002, #4185 ),
 .UNSPECIFIED., .F., .F.,
 ( 4, 2, 2, 2, 2, 2, 2, 2, 2, 2, 2, 2, 2, 2, 2, 2, 2, 2, 2, 2, 2, 2, 2, 2, 2, 2, 2, 2, 2, 2, 2, 2, 2, 2, 2, 4 ),
 ( 0.1589808399053934673, 0.1602572277490322550, 0.1615336155926710426, 0.1628100034363098303, 0.1640863912799486179, 0.1666391669672261933, 0.1691919426545037686, 0.1717447183417813439, 0.1742974940290588914, 0.1794030454036140143, 0.1819558210908915896, 0.1832322089345303495, 0.1845085967781691372, 0.1896141481527242600, 0.1908905359963630199, 0.1921669238400018076, 0.1947196995272793552, 0.1972724752145569305, 0.1998252509018344780, 0.2011016387454732657, 0.2023780265891120256, 0.2049308022763896009, 0.2074835779636671484, 0.2100363536509446960, 0.2125891293382222713, 0.2138655171818610590, 0.2151419050254998466, 0.2202474564000549972, 0.2228002320873325726, 0.2253530077746101479, 0.2304585591491652985, 0.2330113348364428738, 0.2355641105237204491, 0.2368404983673592368, 0.2381168862109980244, 0.2406696618982755997 ),
 .UNSPECIFIED. ) ;
#8359=CARTESIAN_POINT ( 'NONE',  ( -73.90625000204839523, 36.74823131438026280, 18.25176868561974786 ) ) ;
#8369=FACE_OUTER_BOUND ( 'NONE', #5366, .T. ) ;
#8376=CARTESIAN_POINT ( 'NONE',  ( -77.18750000000007105, 37.32233047033638229, -17.67766952966361771 ) ) ;
#8384=DIRECTION ( 'NONE',  ( 0.000000000000000000, 0.000000000000000000, 1.000000000000000000 ) ) ;
#8385=CARTESIAN_POINT ( 'NONE',  ( 3.744923233462341604E-15, 110.0000000000000000, -30.57961884250791940 ) ) ;
#8390=CARTESIAN_POINT ( 'NONE',  ( -75.96875000204839523, 80.81189881250000440, -1.580522963032174394E-15 ) ) ;
#8392=CARTESIAN_POINT ( 'NONE',  ( 25.29007368494098884, 80.00022686158581564, -0.4132073972999723566 ) ) ;
#8394=CARTESIAN_POINT ( 'NONE',  ( -71.34302368722835297, 77.35376350879521112, 12.90594348738575903 ) ) ;
#8395=FACE_BOUND ( 'NONE', #988, .T. ) ;
#8396=CARTESIAN_POINT ( 'NONE',  ( 39.99999999999999289, 55.00000000000000000, 0.000000000000000000 ) ) ;
#8398=LINE ( 'NONE', #10062, #3813 ) ;
#8404=CARTESIAN_POINT ( 'NONE',  ( -14.41642088558921486, 71.22858682633147964, 14.86374956074409681 ) ) ;
#8413=CARTESIAN_POINT ( 'NONE',  ( -72.68750000204839523, 44.30836144126053000, 25.81189881250000795 ) ) ;
#8421=CARTESIAN_POINT ( 'NONE',  ( -72.21875000204838102, 29.18810118750000271, 4.741568889096522788E-15 ) ) ;
#8429=CARTESIAN_POINT ( 'NONE',  ( 14.99999999999999645, -30.00000000000000000, -10.00000000000000000 ) ) ;
#8432=VERTEX_POINT ( 'NONE', #2396 ) ;
#8436=ADVANCED_FACE ( 'NONE', ( #6854 ), #9761, .T. ) ;
#8437=EDGE_CURVE ( 'NONE', #5411, #7145, #6417, .T. ) ;
#8438=DIRECTION ( 'NONE',  ( -0.000000000000000000, -1.000000000000000000, -0.000000000000000000 ) ) ;
#8439=EDGE_CURVE ( 'NONE', #9870, #11, #4261, .T. ) ;
#8449=( BOUNDED_CURVE ( )  B_SPLINE_CURVE ( 2, ( #9350, #9286, #11197, #10305, #11079, #1922, #3007, #7386, #6677 ),
 .UNSPECIFIED., .F., .T. ) 
 B_SPLINE_CURVE_WITH_KNOTS ( ( 3, 2, 2, 2, 3 ),
 ( 0.5545069179274292326, 0.5743159892607880845, 0.5941250605941470475, 0.6139341319275060105, 0.6337432032608648624 ),
 .UNSPECIFIED. ) 
 CURVE ( )  GEOMETRIC_REPRESENTATION_ITEM ( )  RATIONAL_B_SPLINE_CURVE ( ( 1.000000000000015321, 0.9238795325112713064, 1.000000000000000000, 0.9238795325112867385, 1.000000000000000000, 0.9238795325112867385, 1.000000000000000000, 0.9238795325112867385, 1.000000000000000000 ) ) 
 REPRESENTATION_ITEM ( '' )  );
#8450=CARTESIAN_POINT ( 'NONE',  ( -72.03125000204838102, 55.00000000000000000, -25.81189881249999729 ) ) ;
#8453=CARTESIAN_POINT ( 'NONE',  ( -77.18750000409679046, 72.67766952966368876, -17.67766952966368876 ) ) ;
#8457=CARTESIAN_POINT ( 'NONE',  ( 24.47797982529632321, 79.30575909152375402, -5.865156235303714993 ) ) ;
#8462=CARTESIAN_POINT ( 'NONE',  ( -4.067038661182964928E-21, 64.99605696851786263, 19.59792961213366169 ) ) ;
#8463=VECTOR ( 'NONE', #3257, 1000.000000000000000 ) ;
#8464=ORIENTED_EDGE ( 'NONE', *, *, #4044, .F. ) ;
#8467=CARTESIAN_POINT ( 'NONE',  ( -71.38989868722833876, 77.35376350879521112, 12.90594348738575903 ) ) ;
#8468=DIRECTION ( 'NONE',  ( -1.000000000000000000, -0.000000000000000000, -0.000000000000000000 ) ) ;
#8474=CARTESIAN_POINT ( 'NONE',  ( -73.81250000409677625, 72.67766952966368876, 17.67766952966368521 ) ) ;
#8478=CARTESIAN_POINT ( 'NONE',  ( -72.78125000204839523, 73.25176868561975141, 18.25176868561974075 ) ) ;
#8485=CARTESIAN_POINT ( 'NONE',  ( -71.65625000204839523, 73.25176868561975141, -18.25176868561974430 ) ) ;
#8493=CARTESIAN_POINT ( 'NONE',  ( -79.43750000204838102, 55.00000000000000000, -24.99999999999999645 ) ) ;
#8498=FACE_OUTER_BOUND ( 'NONE', #3526, .T. ) ;
#8499=CARTESIAN_POINT ( 'NONE',  ( 14.99999999999999645, 5.000000000000000000, -29.99999999999999289 ) ) ;
#8510=CARTESIAN_POINT ( 'NONE',  ( -73.90625000204839523, 36.74823131438026280, 18.25176868561974786 ) ) ;
#8511=CARTESIAN_POINT ( 'NONE',  ( -78.12500000409677625, 55.00000000000000000, 24.99999999999999645 ) ) ;
#8512=CARTESIAN_POINT ( 'NONE',  ( 8.878302819564396486, 67.93238317198033371, -21.39628370427902126 ) ) ;
#8520=CARTESIAN_POINT ( 'NONE',  ( -75.78125000000001421, 30.00000000000000355, -10.35533905932738108 ) ) ;
#8525=CARTESIAN_POINT ( 'NONE',  ( -13.90763988834204135, 70.86184651638554044, 15.25345997699037426 ) ) ;
#8526=DIRECTION ( 'NONE',  ( 0.000000000000000000, 0.000000000000000000, -1.000000000000000000 ) ) ;
#8529=CARTESIAN_POINT ( 'NONE',  ( -78.40625000204838102, 29.18810118750000271, 4.741568889096522788E-15 ) ) ;
#8533=CARTESIAN_POINT ( 'NONE',  ( -71.75000000204840944, 65.69163855873948421, -25.81189881250000440 ) ) ;
#8534=CIRCLE ( 'NONE', #3745, 30.57961884250791940 ) ;
#8537=CARTESIAN_POINT ( 'NONE',  ( -77.65625000409676204, 30.00000000000000355, -10.35533905932738108 ) ) ;
#8538=STYLED_ITEM('',(#11902),#8858);
#8540=CARTESIAN_POINT ( 'NONE',  ( -71.34302368722833876, 77.35376350879521112, 12.90594348738575903 ) ) ;
#8544=EDGE_LOOP ( 'NONE', ( #9778, #6102, #3477, #3443 ) ) ;
#8547=LINE ( 'NONE', #11397, #7853 ) ;
#8552=CARTESIAN_POINT ( 'NONE',  ( 39.99999999999999289, 55.00000000000000000, 24.99999999999999645 ) ) ;
#8564=EDGE_CURVE ( 'NONE', #11498, #3514, #4714, .T. ) ;
#8571=CARTESIAN_POINT ( 'NONE',  ( -78.87500000409677625, 55.00000000000000000, -24.99999999999999645 ) ) ;
#8573=CARTESIAN_POINT ( 'NONE',  ( 23.34710263473544245, 78.34793618746451216, -8.970954660865723795 ) ) ;
#8577=FACE_OUTER_BOUND ( 'NONE', #6901, .T. ) ;
#8578=DIRECTION ( 'NONE',  ( -0.000000000000000000, -1.000000000000000000, -0.000000000000000000 ) ) ;
#8583=EDGE_CURVE ( 'NONE', #1747, #7962, #10364, .T. ) ;
#8585=CARTESIAN_POINT ( 'NONE',  ( -74.65625000000000000, 44.64466094067262958, 25.00000000000001066 ) ) ;
#8588=CARTESIAN_POINT ( 'NONE',  ( -79.53125000204838102, 55.00000000000000000, -25.81189881249999729 ) ) ;
#8589=EDGE_LOOP ( 'NONE', ( #9342, #2888, #9816, #549 ) ) ;
#8593=CARTESIAN_POINT ( 'NONE',  ( -72.87500000000007105, 30.00000000000014211, 4.592425496802547545E-15 ) ) ;
#8594=( LENGTH_UNIT ( ) NAMED_UNIT ( * ) SI_UNIT ( .MILLI., .METRE. ) );
#8596=EDGE_LOOP ( 'NONE', ( #6867, #1121, #1397, #7746 ) ) ;
#8598=CARTESIAN_POINT ( 'NONE',  ( -76.25000000204838102, 80.81189881250000440, -10.69163855873948954 ) ) ;
#8599=ORIENTED_EDGE ( 'NONE', *, *, #5431, .F. ) ;
#8601=CARTESIAN_POINT ( 'NONE',  ( -71.34302368722833876, 77.35376350879521112, 12.90594348738575903 ) ) ;
#8604=AXIS2_PLACEMENT_3D ( 'NONE', #11099, #7478, #3030 ) ;
#8607=CARTESIAN_POINT ( 'NONE',  ( -73.81250000204839523, 29.18810118750000981, 10.69163855873950020 ) ) ;
#8614=DIRECTION ( 'NONE',  ( -0.000000000000000000, -1.000000000000000000, -0.000000000000000000 ) ) ;
#8615=CARTESIAN_POINT ( 'NONE',  ( -76.43750000409679046, 37.32233047033631124, 17.67766952966369232 ) ) ;
#8626=CARTESIAN_POINT ( 'NONE',  ( -76.53125000204839523, 36.74823131438024859, -18.25176868561973720 ) ) ;
#8628=CARTESIAN_POINT ( 'NONE',  ( -76.15625000000005684, 44.64466094067266511, 24.99999999999990408 ) ) ;
#8632=CARTESIAN_POINT ( 'NONE',  ( -72.31250000204839523, 29.18810118750000981, 10.69163855873950020 ) ) ;
#8635=AXIS2_PLACEMENT_3D ( 'NONE', #7422, #2073, #11048 ) ;
#8639=CARTESIAN_POINT ( 'NONE',  ( -80.00000000000000000, 55.00000000000000000, 0.000000000000000000 ) ) ;
#8643=CARTESIAN_POINT ( 'NONE',  ( -76.81250000000000000, 72.67766952966368876, -17.67766952966368876 ) ) ;
#8648=CARTESIAN_POINT ( 'NONE',  ( -4.067038661182964928E-21, 64.99605696851786263, 19.59792961213366169 ) ) ;
#8652=CARTESIAN_POINT ( 'NONE',  ( 16.74690967851898193, 72.97670680155702883, -12.69534381283042279 ) ) ;
#8653=CARTESIAN_POINT ( 'NONE',  ( -75.50000000204840944, 29.18810118750000981, 10.69163855873950020 ) ) ;
#8657=CARTESIAN_POINT ( 'NONE',  ( -73.53125000204839523, 36.74823131438024859, -18.25176868561973720 ) ) ;
#8676=CARTESIAN_POINT ( 'NONE',  ( -15.00000000000000355, 5.000000000000000000, 30.00000000000000711 ) ) ;
#8679=VERTEX_POINT ( 'NONE', #1027 ) ;
#8682=DIRECTION ( 'NONE',  ( 0.000000000000000000, 0.000000000000000000, -1.000000000000000000 ) ) ;
#8683=CARTESIAN_POINT ( 'NONE',  ( -77.75000000204839523, 65.69163855873948421, -25.81189881250000084 ) ) ;
#8685=CARTESIAN_POINT ( 'NONE',  ( -19.49409276286124637, 75.18365745446243409, 14.82016776532273816 ) ) ;
#8688=CARTESIAN_POINT ( 'NONE',  ( -76.43750000409679046, 37.32233047033631124, 17.67766952966369232 ) ) ;
#8692=CARTESIAN_POINT ( 'NONE',  ( -75.31250000000005684, 72.67766952966361771, -17.67766952966360705 ) ) ;
#8696=ORIENTED_EDGE ( 'NONE', *, *, #5711, .F. ) ;
#8698=CARTESIAN_POINT ( 'NONE',  ( -72.31250000000000000, 72.67766952966368876, -17.67766952966368876 ) ) ;
#8702=ORIENTED_EDGE ( 'NONE', *, *, #4324, .T. ) ;
#8708=CARTESIAN_POINT ( 'NONE',  ( 20.32841434030235561, 75.84512567670806504, 7.042511973064372377 ) ) ;
#8711=CARTESIAN_POINT ( 'NONE',  ( -73.62500000204842365, 29.18810118750000626, -10.69163855873949309 ) ) ;
#8713=CARTESIAN_POINT ( 'NONE',  ( -75.59375000409677625, 80.00000000000001421, -10.35533905932737753 ) ) ;
#8716=VERTEX_POINT ( 'NONE', #5657 ) ;
#8735=EDGE_CURVE ( 'NONE', #10918, #8848, #7021, .T. ) ;
#8740=CARTESIAN_POINT ( 'NONE',  ( -74.28125000204839523, 73.25176868561975141, 18.25176868561974075 ) ) ;
#8741=CARTESIAN_POINT ( 'NONE',  ( -24.47794101355583862, 79.30561927337025452, -5.910399932586783756 ) ) ;
#8744=CARTESIAN_POINT ( 'NONE',  ( -74.93750000409677625, 37.32233047033631124, 17.67766952966369232 ) ) ;
#8749=CARTESIAN_POINT ( 'NONE',  ( -75.12500000000007105, 79.99999999999988631, -1.530808498934184619E-15 ) ) ;
#8752=DIRECTION ( 'NONE',  ( 0.000000000000000000, 0.000000000000000000, 1.000000000000000000 ) ) ;
#8756=CARTESIAN_POINT ( 'NONE',  ( -76.71875000000000000, 80.00000000000001421, -10.35533905932737753 ) ) ;
#8761=( BOUNDED_CURVE ( )  B_SPLINE_CURVE ( 2, ( #1893, #8255, #7425, #5388, #8198, #6406, #11774 ),
 .UNSPECIFIED., .F., .T. ) 
 B_SPLINE_CURVE_WITH_KNOTS ( ( 3, 2, 2, 3 ),
 ( 0.8333333333333340365, 0.8541666666666670737, 0.8750000000000002220, 0.8888490476107191451 ),
 .UNSPECIFIED. ) 
 CURVE ( )  GEOMETRIC_REPRESENTATION_ITEM ( )  RATIONAL_B_SPLINE_CURVE ( ( 0.9999999999999975575, 0.9238795325112891810, 1.000000000000000000, 0.9238795325112867385, 1.000000000000000000, 0.9493985930367334625, 0.9660721903170175207 ) ) 
 REPRESENTATION_ITEM ( '' )  );
#8765=CIRCLE ( 'NONE', #720, 24.99999999999999645 ) ;
#8767=CARTESIAN_POINT ( 'NONE',  ( 3.623988215512224720, 65.45978901809303352, -19.35591671848164097 ) ) ;
#8771=EDGE_CURVE ( 'NONE', #9843, #4769, #10128, .T. ) ;
#8772=LINE ( 'NONE', #8552, #10337 ) ;
#8778=CARTESIAN_POINT ( 'NONE',  ( -15.00000000000000000, 5.000000000000000000, -20.00000000000000000 ) ) ;
#8784=CARTESIAN_POINT ( 'NONE',  ( -74.28125000204838102, 55.00000000000000000, 25.81189881249999729 ) ) ;
#8791=DIRECTION ( 'NONE',  ( -1.000000000000000000, -0.000000000000000000, -0.000000000000000000 ) ) ;
#8793=AXIS2_PLACEMENT_3D ( 'NONE', #7960, #8802, #8914 ) ;
#8801=CARTESIAN_POINT ( 'NONE',  ( -77.65625000204839523, 73.25176868561975141, -18.25176868561974430 ) ) ;
#8802=DIRECTION ( 'NONE',  ( 0.000000000000000000, 1.000000000000000000, 0.000000000000000000 ) ) ;
#8806=ORIENTED_EDGE ( 'NONE', *, *, #6552, .T. ) ;
#8807=CARTESIAN_POINT ( 'NONE',  ( -75.31250000409677625, 72.67766952966368876, 17.67766952966368521 ) ) ;
#8817=CARTESIAN_POINT ( 'NONE',  ( -78.12500000204838102, 44.30836144126050158, -25.81189881249999374 ) ) ;
#8820=CYLINDRICAL_SURFACE ( 'NONE', #8829, 5.249999999999998224 ) ;
#8826=CARTESIAN_POINT ( 'NONE',  ( 0.000000000000000000, 110.0000000000000000, 0.000000000000000000 ) ) ;
#8828=CARTESIAN_POINT ( 'NONE',  ( 21.49960740303508544, 76.81950186437471473, -2.905261289213686204 ) ) ;
#8829=AXIS2_PLACEMENT_3D ( 'NONE', #2401, #8101, #1447 ) ;
#8831=CARTESIAN_POINT ( 'NONE',  ( -72.59375000204838102, 36.74823131438026280, 18.25176868561974786 ) ) ;
#8834=CARTESIAN_POINT ( 'NONE',  ( -79.25000000000000000, 55.00000000000000000, 24.99999999999999645 ) ) ;
#8843=ORIENTED_EDGE ( 'NONE', *, *, #8439, .F. ) ;
#8847=CARTESIAN_POINT ( 'NONE',  ( -78.78125000204838102, 55.00000000000000000, 25.81189881249999729 ) ) ;
#8848=VERTEX_POINT ( 'NONE', #6863 ) ;
#8858=MANIFOLD_SOLID_BREP ( 'AdvancedHole1', #1942 ) ;
#8859=LINE ( 'NONE', #4366, #2602 ) ;
#8864=CARTESIAN_POINT ( 'NONE',  ( -71.56250000409677625, 37.32233047033631124, -17.67766952966368166 ) ) ;
#8875=CARTESIAN_POINT ( 'NONE',  ( -75.12500000204838102, 44.30836144126050158, -25.81189881249999374 ) ) ;
#8877=ORIENTED_EDGE ( 'NONE', *, *, #9211, .F. ) ;
#8878=DIRECTION ( 'NONE',  ( 1.000000000000000000, 0.000000000000000000, 0.000000000000000000 ) ) ;
#8884=CARTESIAN_POINT ( 'NONE',  ( 21.67169741744320888, 76.96394498674538909, -1.454759563390118471 ) ) ;
#8889=DIRECTION ( 'NONE',  ( 0.000000000000000000, 1.000000000000000000, 0.000000000000000000 ) ) ;
#8898=ORIENTED_EDGE ( 'NONE', *, *, #10409, .F. ) ;
#8901=CARTESIAN_POINT ( 'NONE',  ( -79.15625000204838102, 80.81189881250000440, -1.580522963032174394E-15 ) ) ;
#8908=CARTESIAN_POINT ( 'NONE',  ( -70.87427368927673399, 76.65063840437989029, 12.49999426731031704 ) ) ;
#8914=DIRECTION ( 'NONE',  ( 0.000000000000000000, 0.000000000000000000, 1.000000000000000000 ) ) ;
#8917=CARTESIAN_POINT ( 'NONE',  ( -73.90625000409680467, 80.00000000000001421, 10.35533905932737397 ) ) ;
#8919=DIRECTION ( 'NONE',  ( -1.000000000000000000, -0.000000000000000000, -0.000000000000000000 ) ) ;
#8932=CARTESIAN_POINT ( 'NONE',  ( -79.53125000204838102, 55.00000000000000000, -25.81189881249999729 ) ) ;
#8935=AXIS2_PLACEMENT_3D ( 'NONE', #594, #6791, #7856 ) ;
#8936=CARTESIAN_POINT ( 'NONE',  ( -72.12500000409677625, 55.00000000000000000, 24.99999999999999645 ) ) ;
#8938=CARTESIAN_POINT ( 'NONE',  ( 22.80989338617025552, 77.89797702579812722, 10.04169729082317986 ) ) ;
#8941=CARTESIAN_POINT ( 'NONE',  ( -78.59375000000001421, 44.64466094067047663, -24.99999999999782219 ) ) ;
#8942=EDGE_CURVE ( 'NONE', #2575, #6052, #488, .T. ) ;
#8945=CARTESIAN_POINT ( 'NONE',  ( -77.93750000000005684, 72.67766952966363192, 17.67766952966363547 ) ) ;
#8946=CARTESIAN_POINT ( 'NONE',  ( -72.68750000204839523, 44.30836144126052289, 25.81189881250000795 ) ) ;
#8951=CARTESIAN_POINT ( 'NONE',  ( 14.99999999999999645, 5.000000000000000000, 30.00000000000000711 ) ) ;
#8953=EDGE_CURVE ( 'NONE', #8979, #5671, #3543, .T. ) ;
#8964=CARTESIAN_POINT ( 'NONE',  ( -78.40625000204838102, 29.18810118750000271, 4.741568889096522788E-15 ) ) ;
#8970=CARTESIAN_POINT ( 'NONE',  ( 9.999999999999994671, -30.00000000000000000, -10.00000000000000000 ) ) ;
#8976=FACE_OUTER_BOUND ( 'NONE', #6696, .T. ) ;
#8979=VERTEX_POINT ( 'NONE', #7098 ) ;
#8988=CARTESIAN_POINT ( 'NONE',  ( -78.59375000409677625, 80.00000000000001421, -10.35533905932737753 ) ) ;
#8993=CARTESIAN_POINT ( 'NONE',  ( -77.65625000204838102, 80.81189881250000440, -1.580522963032174394E-15 ) ) ;
#9004=CARTESIAN_POINT ( 'NONE',  ( -72.87500000204838102, 65.69163855873949842, 25.81189881250000084 ) ) ;
#9020=CARTESIAN_POINT ( 'NONE',  ( -74.93750000204839523, 65.69163855873948421, -25.81189881250000440 ) ) ;
#9026=SURFACE_SIDE_STYLE ('',( #3454 ) ) ;
#9035=CARTESIAN_POINT ( 'NONE',  ( -75.59375000000005684, 44.64466094067241642, -24.99999999999965539 ) ) ;
#9036=FACE_OUTER_BOUND ( 'NONE', #2961, .T. ) ;
#9048=CARTESIAN_POINT ( 'NONE',  ( -74.18750000204838102, 44.30836144126053000, 25.81189881250000795 ) ) ;
#9051=CARTESIAN_POINT ( 'NONE',  ( -75.21875000204839523, 29.18810118750000271, 4.741568889096522788E-15 ) ) ;
#9053=CARTESIAN_POINT ( 'NONE',  ( 4.235829868893991268, 66.01841521325340523, 22.44289296408692991 ) ) ;
#9057=CARTESIAN_POINT ( 'NONE',  ( 1.474044695502842117, 65.07161681208872039, -19.55923518678806161 ) ) ;
#9058=EDGE_LOOP ( 'NONE', ( #8185, #4798 ) ) ;
#9069=EDGE_LOOP ( 'NONE', ( #5961, #1283 ) ) ;
#9073=VERTEX_POINT ( 'NONE', #6313 ) ;
#9075=CARTESIAN_POINT ( 'NONE',  ( -72.96875000204838102, 73.25176868561975141, 18.25176868561974075 ) ) ;
#9080=LINE ( 'NONE', #8970, #3235 ) ;
#9081=EDGE_CURVE ( 'NONE', #9521, #7673, #1261, .T. ) ;
#9083=ORIENTED_EDGE ( 'NONE', *, *, #11821, .T. ) ;
#9085=EDGE_CURVE ( 'NONE', #6717, #193, #10738, .T. ) ;
#9102=CARTESIAN_POINT ( 'NONE',  ( -73.90625000204838102, 29.18810118750000271, 4.741568889096522788E-15 ) ) ;
#9106=CARTESIAN_POINT ( 'NONE',  ( -75.50000000204840944, 44.30836144126053000, 25.81189881250000795 ) ) ;
#9108=CARTESIAN_POINT ( 'NONE',  ( 17.59011022552445880, 73.70148073974591796, 16.59389287537950963 ) ) ;
#9111=CARTESIAN_POINT ( 'NONE',  ( 39.99999999999999289, 55.00000000000000000, -24.99999999999999645 ) ) ;
#9115=DIRECTION ( 'NONE',  ( 0.000000000000000000, 0.000000000000000000, 1.000000000000000000 ) ) ;
#9117=LINE ( 'NONE', #1, #3647 ) ;
#9119=PRODUCT_CONTEXT ( 'NONE', #5325, 'mechanical' ) ;
#9120=CARTESIAN_POINT ( 'NONE',  ( -17.17085726908380394, 73.30622707836364782, -12.21665692408397241 ) ) ;
#9124=VERTEX_POINT ( 'NONE', #4391 ) ;
#9129=CARTESIAN_POINT ( 'NONE',  ( -72.03125000204838102, 55.00000000000000000, -25.81189881249999729 ) ) ;
#9135=EDGE_CURVE ( 'NONE', #193, #8038, #50, .T. ) ;
#9144=CARTESIAN_POINT ( 'NONE',  ( -72.96875000409677625, 44.64466094067281432, -25.00000000000019540 ) ) ;
#9153=CARTESIAN_POINT ( 'NONE',  ( -78.21875000409677625, 65.35533905932734910, 25.00000000000002132 ) ) ;
#9158=DIRECTION ( 'NONE',  ( -1.000000000000000000, -0.000000000000000000, -0.000000000000000000 ) ) ;
#9160=CARTESIAN_POINT ( 'NONE',  ( -20.20056265816597829, 75.75497107137435648, -13.94119571728393225 ) ) ;
#9168=ADVANCED_FACE ( 'NONE', ( #8395, #954 ), #4866, .T. ) ;
#9172=AXIS2_PLACEMENT_3D ( 'NONE', #9978, #1774, #5440 ) ;
#9174=ORIENTED_EDGE ( 'NONE', *, *, #3084, .F. ) ;
#9175=CARTESIAN_POINT ( 'NONE',  ( -79.71875000000001421, 80.00000000000001421, -10.35533905932737753 ) ) ;
#9177=CYLINDRICAL_SURFACE ( 'NONE', #9766, 24.99999999999999645 ) ;
#9181=CARTESIAN_POINT ( 'NONE',  ( -21.27969014566767569, 76.63537834043187047, -4.004875479550875639 ) ) ;
#9187=CARTESIAN_POINT ( 'NONE',  ( -72.78125000204838102, 55.00000000000000000, 25.81189881249999729 ) ) ;
#9201=B_SPLINE_CURVE_WITH_KNOTS ( 'NONE', 3,
 ( #8224, #2825, #4810, #6559 ),
 .UNSPECIFIED., .F., .F.,
 ( 4, 4 ),
 ( 0.000000000000000000, 1.000000000000000000 ),
 .UNSPECIFIED. ) ;
#9205=LINE ( 'NONE', #4654, #7099 ) ;
#9207=( BOUNDED_CURVE ( )  B_SPLINE_CURVE ( 2, ( #1781, #2751, #10041, #3825, #7491, #4905, #8376, #10344, #10284 ),
 .UNSPECIFIED., .F., .T. ) 
 B_SPLINE_CURVE_WITH_KNOTS ( ( 3, 2, 2, 2, 3 ),
 ( 0.2376281879409543607, 0.2574394709827818040, 0.2772507540246093027, 0.2970620370664368015, 0.3168733201082642448 ),
 .UNSPECIFIED. ) 
 CURVE ( )  GEOMETRIC_REPRESENTATION_ITEM ( )  RATIONAL_B_SPLINE_CURVE ( ( 0.9999999999999494849, 0.9238795325113373647, 1.000000000000000000, 0.9238795325112868495, 1.000000000000000000, 0.9238795325112868495, 1.000000000000000000, 0.9238795325112868495, 1.000000000000000000 ) ) 
 REPRESENTATION_ITEM ( '' )  );
#9208=CARTESIAN_POINT ( 'NONE',  ( -76.25000000000000000, 55.00000000000000000, 24.99999999999999645 ) ) ;
#9211=EDGE_CURVE ( 'NONE', #2686, #4040, #8275, .T. ) ;
#9214=CARTESIAN_POINT ( 'NONE',  ( -78.50000000409677625, 80.00000000000000000, -1.530808498934191324E-15 ) ) ;
#9217=CARTESIAN_POINT ( 'NONE',  ( -72.40625000204838102, 29.18810118750000271, 4.741568889096522788E-15 ) ) ;
#9218=CARTESIAN_POINT ( 'NONE',  ( 0.000000000000000000, 110.0000000000000000, 0.000000000000000000 ) ) ;
#9220=CARTESIAN_POINT ( 'NONE',  ( -72.59375000204838102, 36.74823131438026280, 18.25176868561974786 ) ) ;
#9225=( NAMED_UNIT ( * ) SI_UNIT ( $, .STERADIAN. ) SOLID_ANGLE_UNIT ( ) );
#9232=CARTESIAN_POINT ( 'NONE',  ( 2.087481099544137350E-15, 50.52094453300079380, -17.04557674096337649 ) ) ;
#9239=CARTESIAN_POINT ( 'NONE',  ( -19.09301521363747511, 74.83539102382144392, -9.521771482395543273 ) ) ;
#9247=CARTESIAN_POINT ( 'NONE',  ( -79.06250000204840944, 80.81189881250001861, -10.69163855873949132 ) ) ;
#9251=ORIENTED_EDGE ( 'NONE', *, *, #8735, .F. ) ;
#9253=CARTESIAN_POINT ( 'NONE',  ( -71.84375000204838102, 55.00000000000000000, -25.81189881249999729 ) ) ;
#9254=CARTESIAN_POINT ( 'NONE',  ( -72.40625000409679046, 80.00000000000001421, 10.35533905932737397 ) ) ;
#9260=FACE_OUTER_BOUND ( 'NONE', #9681, .T. ) ;
#9273=CARTESIAN_POINT ( 'NONE',  ( -11.01335487196557850, 69.13152664304863038, -20.62949354447422223 ) ) ;
#9277=CARTESIAN_POINT ( 'NONE',  ( -78.78125000204839523, 73.25176868561975141, 18.25176868561974075 ) ) ;
#9278=VERTEX_POINT ( 'NONE', #10535 ) ;
#9286=CARTESIAN_POINT ( 'NONE',  ( -74.65625000000008527, 44.64466094067429225, 25.00000000000147082 ) ) ;
#9292=CARTESIAN_POINT ( 'NONE',  ( -20.34731364127066655, 75.86048710458229039, 7.023288102819432055 ) ) ;
#9294=EDGE_CURVE ( 'NONE', #896, #4200, #9502, .T. ) ;
#9298=CARTESIAN_POINT ( 'NONE',  ( 14.99999999999999289, 39.99999999999999289, 19.99999999999999289 ) ) ;
#9302=CARTESIAN_POINT ( 'NONE',  ( -71.93750000204838102, 65.69163855873948421, -25.81189881250000440 ) ) ;
#9307=LINE ( 'NONE', #4761, #7504 ) ;
#9309=VECTOR ( 'NONE', #3843, 1000.000000000000000 ) ;
#9320=CARTESIAN_POINT ( 'NONE',  ( -73.06250000409677625, 37.32233047033631124, -17.67766952966368166 ) ) ;
#9334=DIRECTION ( 'NONE',  ( 0.000000000000000000, 0.000000000000000000, 1.000000000000000000 ) ) ;
#9337=CARTESIAN_POINT ( 'NONE',  ( -21.39751393901811838, 76.72268714209511131, -12.45540278537336754 ) ) ;
#9341=CARTESIAN_POINT ( 'NONE',  ( -73.81250000204839523, 29.18810118750000981, 10.69163855873950020 ) ) ;
#9342=ORIENTED_EDGE ( 'NONE', *, *, #7566, .F. ) ;
#9343=CARTESIAN_POINT ( 'NONE',  ( 25.08633069608793420, 79.82547947451034531, 2.979094639268365263 ) ) ;
#9350=CARTESIAN_POINT ( 'NONE',  ( -74.75000000000000000, 55.00000000000000000, 24.99999999999999645 ) ) ;
#9354=PLANE ( 'NONE',  #2284 ) ;
#9371=EDGE_CURVE ( 'NONE', #5671, #1709, #6965, .T. ) ;
#9372=CARTESIAN_POINT ( 'NONE',  ( -72.78125000409680467, 65.35533905932757648, -24.99999999999979039 ) ) ;
#9393=ORIENTED_EDGE ( 'NONE', *, *, #9466, .T. ) ;
#9398=CARTESIAN_POINT ( 'NONE',  ( -25.28844287072157471, 79.99882686206473181, -0.8862795495640891641 ) ) ;
#9401=CARTESIAN_POINT ( 'NONE',  ( -73.71875000204839523, 29.18810118750000271, 4.741568889096522788E-15 ) ) ;
#9404=CARTESIAN_POINT ( 'NONE',  ( 25.28926814670273515, 79.99953533380057991, 0.8669296567843869372 ) ) ;
#9410=VECTOR ( 'NONE', #4277, 1000.000000000000000 ) ;
#9418=CARTESIAN_POINT ( 'NONE',  ( -0.7331957588256760028, 64.99605696851789105, 19.59792961213366880 ) ) ;
#9424=ORIENTED_EDGE ( 'NONE', *, *, #2586, .F. ) ;
#9426=CARTESIAN_POINT ( 'NONE',  ( -72.12500000204840944, 29.18810118750000626, -10.69163855873949309 ) ) ;
#9427=CARTESIAN_POINT ( 'NONE',  ( -1.625240267017640655E-20, 65.42943686846950868, 22.72062601704910634 ) ) ;
#9443=ADVANCED_FACE ( 'NONE', ( #9818, #1729 ), #8094, .T. ) ;
#9445=CARTESIAN_POINT ( 'NONE',  ( -15.00000000000000000, -30.00000000000000000, 10.00000000000000000 ) ) ;
#9446=CARTESIAN_POINT ( 'NONE',  ( -79.34375000204839523, 55.00000000000000000, -25.81189881249999729 ) ) ;
#9448=EDGE_CURVE ( 'NONE', #5671, #4962, #2577, .T. ) ;
#9457=CARTESIAN_POINT ( 'NONE',  ( 39.99999999999999289, 55.00000000000000000, 0.000000000000000000 ) ) ;
#9459=CARTESIAN_POINT ( 'NONE',  ( -25.27843518572107229, 79.99023359000550215, 0.8195747360922619462 ) ) ;
#9463=CARTESIAN_POINT ( 'NONE',  ( -71.56250000204838102, 80.81189881250001861, -10.69163855873949132 ) ) ;
#9465=CARTESIAN_POINT ( 'NONE',  ( 5.841383071459858023, 66.54671248543735373, -22.17569923478663796 ) ) ;
#9466=EDGE_CURVE ( 'NONE', #9124, #10874, #4347, .T. ) ;
#9473=CARTESIAN_POINT ( 'NONE',  ( -75.21875000000000000, 80.00000000000001421, -10.35533905932737753 ) ) ;
#9479=CARTESIAN_POINT ( 'NONE',  ( -73.15625000000008527, 44.64466094067268642, 24.99999999999986144 ) ) ;
#9483=CARTESIAN_POINT ( 'NONE',  ( -76.90625000204838102, 29.18810118750000271, 4.741568889096522788E-15 ) ) ;
#9486=CARTESIAN_POINT ( 'NONE',  ( -73.71875000204839523, 29.18810118750000271, 4.741568889096522788E-15 ) ) ;
#9495=EDGE_CURVE ( 'NONE', #8038, #30, #5865, .T. ) ;
#9502=CIRCLE ( 'NONE', #8935, 24.99999999999999645 ) ;
#9504=ORIENTED_EDGE ( 'NONE', *, *, #2939, .T. ) ;
#9516=LINE ( 'NONE', #7729, #10399 ) ;
#9517=CARTESIAN_POINT ( 'NONE',  ( -76.15625000204839523, 73.25176868561975141, -18.25176868561974430 ) ) ;
#9519=CARTESIAN_POINT ( 'NONE',  ( -76.25000000000000000, 55.00000000000000000, 24.99999999999999645 ) ) ;
#9521=VERTEX_POINT ( 'NONE', #939 ) ;
#9523=CARTESIAN_POINT ( 'NONE',  ( -71.65625000204839523, 73.25176868561975141, -18.25176868561974430 ) ) ;
#9526=MECHANICAL_DESIGN_GEOMETRIC_PRESENTATION_REPRESENTATION('',(#5128),#11803);
#9528=CARTESIAN_POINT ( 'NONE',  ( -71.40552368722833876, 77.35376350879521112, 12.90594348738575903 ) ) ;
#9534=CARTESIAN_POINT ( 'NONE',  ( -72.59375000000000000, 44.64466094067260826, -24.99999999999998934 ) ) ;
#9543=ORIENTED_EDGE ( 'NONE', *, *, #4024, .F. ) ;
#9544=CARTESIAN_POINT ( 'NONE',  ( 19.13861104931596202, 74.87002429251506896, 9.536576732248796873 ) ) ;
#9545=CARTESIAN_POINT ( 'NONE',  ( -79.34375000204839523, 73.25176868561975141, -18.25176868561974430 ) ) ;
#9549=CARTESIAN_POINT ( 'NONE',  ( -75.68750000204839523, 65.69163855873949842, 25.81189881250000440 ) ) ;
#9550=CARTESIAN_POINT ( 'NONE',  ( -75.21875000409676204, 65.35533905932724963, 25.00000000000012434 ) ) ;
#9571=CARTESIAN_POINT ( 'NONE',  ( 14.99999999999999645, 5.000000000000000000, 30.00000000000000711 ) ) ;
#9573=VERTEX_POINT ( 'NONE', #2806 ) ;
#9576=CARTESIAN_POINT ( 'NONE',  ( 39.99999999999999289, 39.99999999999999289, 19.99999999999999289 ) ) ;
#9578=CARTESIAN_POINT ( 'NONE',  ( -74.75000000204839523, 65.69163855873948421, -25.81189881250000084 ) ) ;
#9579=CARTESIAN_POINT ( 'NONE',  ( -23.35334274943035737, 78.35318589264019806, 8.957355889116216829 ) ) ;
#9583=CARTESIAN_POINT ( 'NONE',  ( -72.50000000204839523, 44.30836144126053000, 25.81189881250000795 ) ) ;
#9591=ORIENTED_EDGE ( 'NONE', *, *, #64, .T. ) ;
#9594=VECTOR ( 'NONE', #367, 1000.000000000000000 ) ;
#9595=CARTESIAN_POINT ( 'NONE',  ( -76.06250000000000000, 37.32233047033631124, 17.67766952966369232 ) ) ;
#9602=CARTESIAN_POINT ( 'NONE',  ( -6.995124206613962947, 66.69163081399298676, 18.63899971507076003 ) ) ;
#9607=CARTESIAN_POINT ( 'NONE',  ( 12.88440744682079497, 70.13069922856422522, -15.99938705239769021 ) ) ;
#9608=CARTESIAN_POINT ( 'NONE',  ( -77.09375000204839523, 36.74823131438026280, 18.25176868561974786 ) ) ;
#9610=CARTESIAN_POINT ( 'NONE',  ( -72.87500000204840944, 80.81189881250001861, 10.69163855873948599 ) ) ;
#9622=DIRECTION ( 'NONE',  ( -1.000000000000000000, -0.000000000000000000, -0.000000000000000000 ) ) ;
#9634=CARTESIAN_POINT ( 'NONE',  ( -77.37500000204838102, 80.81189881250000440, 10.69163855873948243 ) ) ;
#9635=CARTESIAN_POINT ( 'NONE',  ( -18.44673231479036701, 74.35351539244358321, 15.87705593169374474 ) ) ;
#9638=CARTESIAN_POINT ( 'NONE',  ( -74.46875000409679046, 44.64466094067260826, -24.99999999999998934 ) ) ;
#9649=CARTESIAN_POINT ( 'NONE',  ( -73.81250000000000000, 72.67766952966368876, -17.67766952966368876 ) ) ;
#9658=CARTESIAN_POINT ( 'NONE',  ( 21.03248180003672729, 76.42892261394429454, -5.031022656301434637 ) ) ;
#9659=CARTESIAN_POINT ( 'NONE',  ( -78.68750000204838102, 44.30836144126052289, 25.81189881250000795 ) ) ;
#9662=DIRECTION ( 'NONE',  ( -1.000000000000000000, -0.000000000000000000, -0.000000000000000000 ) ) ;
#9671=EDGE_CURVE ( 'NONE', #9742, #4746, #11508, .T. ) ;
#9681=EDGE_LOOP ( 'NONE', ( #5756, #5739, #3746, #2703 ) ) ;
#9692=CARTESIAN_POINT ( 'NONE',  ( -76.25000000204838102, 65.69163855873948421, -25.81189881250000084 ) ) ;
#9696=CARTESIAN_POINT ( 'NONE',  ( -73.71875000409677625, 65.35533905932737753, 24.99999999999999645 ) ) ;
#9703=DIRECTION ( 'NONE',  ( 1.000000000000000000, 0.000000000000000000, 0.000000000000000000 ) ) ;
#9706=CARTESIAN_POINT ( 'NONE',  ( -74.00000000000000000, 55.00000000000000000, -24.99999999999999645 ) ) ;
#9715=CARTESIAN_POINT ( 'NONE',  ( 20.82503005121913731, 76.25610946991470485, 5.714993128054450366 ) ) ;
#9716=CARTESIAN_POINT ( 'NONE',  ( -73.25000000204838102, 80.81189881250000440, -10.69163855873948954 ) ) ;
#9730=CARTESIAN_POINT ( 'NONE',  ( -79.43750000204838102, 65.69163855873948421, -25.81189881250000440 ) ) ;
#9733=EDGE_LOOP ( 'NONE', ( #4736, #6684 ) ) ;
#9742=VERTEX_POINT ( 'NONE', #3942 ) ;
#9744=CARTESIAN_POINT ( 'NONE',  ( -15.00000000000000355, 0.000000000000000000, -29.99999999999999289 ) ) ;
#9747=CYLINDRICAL_SURFACE ( 'NONE', #1130, 24.99999999999999645 ) ;
#9749=ORIENTED_EDGE ( 'NONE', *, *, #3285, .T. ) ;
#9750=CARTESIAN_POINT ( 'NONE',  ( -71.18750000409677625, 72.67766952966368876, -17.67766952966368876 ) ) ;
#9757=CARTESIAN_POINT ( 'NONE',  ( -15.00000000000000000, -24.99999999999999645, 10.00000000000000000 ) ) ;
#9759=AXIS2_PLACEMENT_3D ( 'NONE', #10045, #9158, #8384 ) ;
#9761=CYLINDRICAL_SURFACE ( 'NONE', #10922, 24.99999999999999645 ) ;
#9762=CARTESIAN_POINT ( 'NONE',  ( -78.78125000204838102, 55.00000000000000000, 25.81189881249999729 ) ) ;
#9766=AXIS2_PLACEMENT_3D ( 'NONE', #1021, #6617, #10961 ) ;
#9768=ADVANCED_FACE ( 'NONE', ( #11234, #7777 ), #5869, .T. ) ;
#9771=CARTESIAN_POINT ( 'NONE',  ( 9.999999999999994671, 0.000000000000000000, 10.00000000000000000 ) ) ;
#9774=CARTESIAN_POINT ( 'NONE',  ( 21.36699128324961805, 76.70829236948175378, 3.640766976057809856 ) ) ;
#9778=ORIENTED_EDGE ( 'NONE', *, *, #1054, .F. ) ;
#9793=CARTESIAN_POINT ( 'NONE',  ( -79.06250000204839523, 80.81189881250001861, 10.69163855873948599 ) ) ;
#9816=ORIENTED_EDGE ( 'NONE', *, *, #9081, .T. ) ;
#9818=FACE_BOUND ( 'NONE', #6411, .T. ) ;
#9824=CARTESIAN_POINT ( 'NONE',  ( -80.00000000000000000, 55.00000000000000000, -24.99999999999999645 ) ) ;
#9825=CARTESIAN_POINT ( 'NONE',  ( -75.50000000204840944, 29.18810118750000981, 10.69163855873950020 ) ) ;
#9833=CARTESIAN_POINT ( 'NONE',  ( -70.87427368927673399, 76.65063840437989029, 12.49999426731031704 ) ) ;
#9834=CARTESIAN_POINT ( 'NONE',  ( -76.62500000409677625, 55.00000000000000000, 24.99999999999999645 ) ) ;
#9836=CARTESIAN_POINT ( 'NONE',  ( -73.43750000204839523, 65.69163855873948421, -25.81189881250000084 ) ) ;
#9843=VERTEX_POINT ( 'NONE', #279 ) ;
#9845=DIRECTION ( 'NONE',  ( 0.000000000000000000, 0.000000000000000000, 1.000000000000000000 ) ) ;
#9846=ORIENTED_EDGE ( 'NONE', *, *, #3169, .F. ) ;
#9848=CARTESIAN_POINT ( 'NONE',  ( -75.87500000204839523, 65.69163855873949842, 25.81189881250000440 ) ) ;
#9853=DIRECTION ( 'NONE',  ( 0.000000000000000000, 1.000000000000000000, 0.000000000000000000 ) ) ;
#9861=CARTESIAN_POINT ( 'NONE',  ( 6.123233995736766282E-16, -24.99999999999999645, 5.000000000000000000 ) ) ;
#9865=CARTESIAN_POINT ( 'NONE',  ( -71.28125000409677625, 65.35533905932737753, -24.99999999999999645 ) ) ;
#9867=CARTESIAN_POINT ( 'NONE',  ( -71.75000000409677625, 30.00000000000000355, 4.592425496802573578E-15 ) ) ;
#9868=VECTOR ( 'NONE', #6836, 1000.000000000000000 ) ;
#9870=VERTEX_POINT ( 'NONE', #8499 ) ;
#9872=CARTESIAN_POINT ( 'NONE',  ( -78.87500000409677625, 55.00000000000000000, -24.99999999999999645 ) ) ;
#9876=CARTESIAN_POINT ( 'NONE',  ( -71.91717626682689968, 72.42551787026226862, 19.81812247078860523 ) ) ;
#9881=VERTEX_POINT ( 'NONE', #10347 ) ;
#9885=ADVANCED_FACE ( 'NONE', ( #5031 ), #3162, .F. ) ;
#9889=CIRCLE ( 'NONE', #7616, 5.249999999999998224 ) ;
#9896=EDGE_CURVE ( 'NONE', #3359, #8432, #4157, .T. ) ;
#9908=CARTESIAN_POINT ( 'NONE',  ( -76.25000000204838102, 80.81189881250001861, -10.69163855873949132 ) ) ;
#9926=CARTESIAN_POINT ( 'NONE',  ( 39.99999999999999289, 55.00000000000000000, -24.99999999999999645 ) ) ;
#9938=CARTESIAN_POINT ( 'NONE',  ( -79.06250000204839523, 80.81189881250001861, 10.69163855873948599 ) ) ;
#9942=CARTESIAN_POINT ( 'NONE',  ( -76.15625000204839523, 73.25176868561975141, -18.25176868561974430 ) ) ;
#9944=CARTESIAN_POINT ( 'NONE',  ( 0.8592290948358244362, 65.44860072268932072, 22.71185887947197557 ) ) ;
#9948=CARTESIAN_POINT ( 'NONE',  ( 0.3675172377051636463, 64.99605696851787684, -19.59792961213366169 ) ) ;
#9949=CARTESIAN_POINT ( 'NONE',  ( -73.15625000204838102, 80.81189881250000440, -1.580522963032174394E-15 ) ) ;
#9958=VECTOR ( 'NONE', #6179, 1000.000000000000000 ) ;
#9964=CARTESIAN_POINT ( 'NONE',  ( -75.40625000204838102, 29.18810118750000271, 4.741568889096522788E-15 ) ) ;
#9965=VECTOR ( 'NONE', #2984, 1000.000000000000000 ) ;
#9967=VERTEX_POINT ( 'NONE', #8908 ) ;
#9973=FACE_OUTER_BOUND ( 'NONE', #9733, .T. ) ;
#9978=CARTESIAN_POINT ( 'NONE',  ( 39.99999999999999289, 55.00000000000000000, 0.000000000000000000 ) ) ;
#9980=ADVANCED_BREP_SHAPE_REPRESENTATION ( '', ( #8858, #4738 ), #3015 ) ;
#9989=VERTEX_POINT ( 'NONE', #11328 ) ;
#9990=CARTESIAN_POINT ( 'NONE',  ( -72.50000000000000000, 55.00000000000000000, -24.99999999999999645 ) ) ;
#9993=CARTESIAN_POINT ( 'NONE',  ( -72.12500000204839523, 44.30836144126050158, -25.81189881249999374 ) ) ;
#9995=ORIENTED_EDGE ( 'NONE', *, *, #7486, .F. ) ;
#9996=CARTESIAN_POINT ( 'NONE',  ( -77.09375000204839523, 55.00000000000000000, 25.81189881249999729 ) ) ;
#10001=EDGE_CURVE ( 'NONE', #10874, #9124, #6855, .T. ) ;
#10010=CARTESIAN_POINT ( 'NONE',  ( -2.541277572167694121, 65.22933659532863260, -19.47729156647515936 ) ) ;
#10018=CARTESIAN_POINT ( 'NONE',  ( -72.50000000204839523, 29.18810118750000981, 10.69163855873950020 ) ) ;
#10033=CARTESIAN_POINT ( 'NONE',  ( 0.000000000000000000, 50.52094453300079380, 17.04557674096337649 ) ) ;
#10036=ADVANCED_FACE ( 'NONE', ( #191 ), #5725, .T. ) ;
#10041=CARTESIAN_POINT ( 'NONE',  ( -77.56250000000007105, 37.32233047033638229, 17.67766952966362837 ) ) ;
#10045=CARTESIAN_POINT ( 'NONE',  ( 39.99999999999999289, 55.00000000000000000, 0.000000000000000000 ) ) ;
#10050=ORIENTED_EDGE ( 'NONE', *, *, #1881, .F. ) ;
#10051=CARTESIAN_POINT ( 'NONE',  ( -74.28125000204839523, 73.25176868561975141, 18.25176868561974075 ) ) ;
#10056=DIRECTION ( 'NONE',  ( 0.000000000000000000, 0.000000000000000000, -1.000000000000000000 ) ) ;
#10059=CARTESIAN_POINT ( 'NONE',  ( -78.21875000000004263, 79.99999999999992895, -10.35533905932734910 ) ) ;
#10061=AXIS2_PLACEMENT_3D ( 'NONE', #9757, #5395, #11730 ) ;
#10062=CARTESIAN_POINT ( 'NONE',  ( 9.999999999999994671, 0.000000000000000000, 10.00000000000000000 ) ) ;
#10066=CARTESIAN_POINT ( 'NONE',  ( -21.53847754367192380, 76.85212920633969702, -2.572070869066138687 ) ) ;
#10068=CARTESIAN_POINT ( 'NONE',  ( 14.99999999999999645, -30.00000000000000000, 10.00000000000000000 ) ) ;
#10071=CARTESIAN_POINT ( 'NONE',  ( -74.37500000409677625, 55.00000000000000000, -24.99999999999999645 ) ) ;
#10074=CARTESIAN_POINT ( 'NONE',  ( -77.93750000204838102, 44.30836144126050158, -25.81189881249999374 ) ) ;
#10075=EDGE_CURVE ( 'NONE', #8154, #9967, #11087, .T. ) ;
#10092=DIRECTION ( 'NONE',  ( -0.000000000000000000, -0.000000000000000000, 1.000000000000000000 ) ) ;
#10095=DIRECTION ( 'NONE',  ( -0.000000000000000000, -1.000000000000000000, -0.000000000000000000 ) ) ;
#10106=CARTESIAN_POINT ( 'NONE',  ( -23.15625510892966687, 78.18806447604573862, -9.352364031898828145 ) ) ;
#10109=CARTESIAN_POINT ( 'NONE',  ( -78.12500000204838102, 29.18810118750000626, -10.69163855873949309 ) ) ;
#10112=CARTESIAN_POINT ( 'NONE',  ( 22.61952844766377169, 77.73902299693440909, 10.39627090682546928 ) ) ;
#10121=CARTESIAN_POINT ( 'NONE',  ( -79.53125000000000000, 80.00000000000001421, 10.35533905932737397 ) ) ;
#10127=CARTESIAN_POINT ( 'NONE',  ( 2.400054171417768487E-15, 64.99605696851786263, -19.59792961213366169 ) ) ;
#10128=LINE ( 'NONE', #4754, #109 ) ;
#10129=VERTEX_POINT ( 'NONE', #9298 ) ;
#10135=CARTESIAN_POINT ( 'NONE',  ( -77.00000000204838102, 44.30836144126053000, 25.81189881250000795 ) ) ;
#10144=CIRCLE ( 'NONE', #7113, 22.00000000000000000 ) ;
#10162=VECTOR ( 'NONE', #841, 1000.000000000000000 ) ;
#10172=CARTESIAN_POINT ( 'NONE',  ( -71.53052369147286527, 77.35376373433385311, 12.90594309674112949 ) ) ;
#10174=EDGE_CURVE ( 'NONE', #8848, #10918, #9889, .T. ) ;
#10180=CARTESIAN_POINT ( 'NONE',  ( 2.782474192756827142E-15, 65.42943686846950868, -22.72062601704910634 ) ) ;
#10184=EDGE_CURVE ( 'NONE', #10529, #2054, #10201, .T. ) ;
#10191=DIRECTION ( 'NONE',  ( -0.000000000000000000, -1.000000000000000000, -0.000000000000000000 ) ) ;
#10192=CARTESIAN_POINT ( 'NONE',  ( -15.00000000000000000, 55.00000000000000000, -20.00000000000000000 ) ) ;
#10194=CARTESIAN_POINT ( 'NONE',  ( -21.48451911196086073, 76.80686963222734676, -2.931110701500045046 ) ) ;
#10201=B_SPLINE_CURVE_WITH_KNOTS ( 'NONE', 3,
 ( #5060, #6865, #1572, #3252, #11505, #6980, #7985, #7750, #11563, #10602, #1339, #611, #2408, #7931, #6081, #4092, #10489, #11384, #9544, #4212, #5970, #8708, #1398, #9715, #5237, #9774, #10554, #1511, #11624, #492, #2354, #6023, #8884, #8828, #7811, #9658, #664, #2295, #5175, #4334, #5001, #4273, #8652, #5901, #3365, #3425, #9607, #1456, #431, #3192, #7041, #2472, #10430, #4147, #5118, #11442, #6922, #8767, #547, #778, #9057, #1624, #9948, #10842 ),
 .UNSPECIFIED., .F., .F.,
 ( 4, 2, 2, 2, 2, 2, 2, 2, 2, 2, 2, 2, 2, 2, 2, 2, 2, 2, 2, 2, 2, 2, 2, 2, 2, 2, 2, 2, 2, 2, 2, 4 ),
 ( 0.1342163981613174739, 0.1363961341890387868, 0.1385758702167600998, 0.1407556062444813849, 0.1429353422722026978, 0.1472948143276453237, 0.1494745503553666088, 0.1516542863830879218, 0.1560137584385305476, 0.1603732304939732012, 0.1614630985078338576, 0.1625529665216945141, 0.1647327025494158825, 0.1669124385771372232, 0.1680023065909978797, 0.1690921746048585639, 0.1712719106325799046, 0.1734516466603012175, 0.1756313826880225581, 0.1778111187157438988, 0.1821705907711865802, 0.1843503267989079208, 0.1865300628266292615, 0.1908895348820719151, 0.1930692709097932558, 0.1952490069375145687, 0.1974287429652359094, 0.1985186109790965658, 0.1996084789929572501, 0.2017882150206785630, 0.2028780830345392472, 0.2039679510483999314 ),
 .UNSPECIFIED. ) ;
#10202=CARTESIAN_POINT ( 'NONE',  ( -74.09375000204839523, 36.74823131438026280, 18.25176868561974786 ) ) ;
#10210=CARTESIAN_POINT ( 'NONE',  ( 0.000000000000000000, 50.52094453300079380, 0.000000000000000000 ) ) ;
#10214=CARTESIAN_POINT ( 'NONE',  ( -73.53125000409677625, 44.64466094067245905, 24.99999999999983658 ) ) ;
#10223=CARTESIAN_POINT ( 'NONE',  ( 9.999999999999994671, -30.00000000000000000, 10.00000000000000000 ) ) ;
#10224=CARTESIAN_POINT ( 'NONE',  ( -78.40625000409677625, 80.00000000000001421, 10.35533905932737397 ) ) ;
#10228=FACE_OUTER_BOUND ( 'NONE', #8544, .T. ) ;
#10230=CARTESIAN_POINT ( 'NONE',  ( -79.25000000204839523, 65.69163855873948421, -25.81189881250000084 ) ) ;
#10231=CARTESIAN_POINT ( 'NONE',  ( -2.993446321628384865, 65.73059443587099793, -22.58010246442618296 ) ) ;
#10234=CARTESIAN_POINT ( 'NONE',  ( -78.68750000409679046, 72.67766952966368876, -17.67766952966368876 ) ) ;
#10236=CARTESIAN_POINT ( 'NONE',  ( 14.31283626472151482, 71.29068060248663130, -18.97189842681568805 ) ) ;
#10250=VECTOR ( 'NONE', #3090, 1000.000000000000000 ) ;
#10255=LINE ( 'NONE', #10, #4996 ) ;
#10259=CARTESIAN_POINT ( 'NONE',  ( -71.46875000204838102, 80.81189881250000440, -1.580522963032174394E-15 ) ) ;
#10266=ORIENTED_EDGE ( 'NONE', *, *, #1168, .T. ) ;
#10267=CARTESIAN_POINT ( 'NONE',  ( -72.68750000204839523, 65.69163855873949842, 25.81189881250000084 ) ) ;
#10274=CARTESIAN_POINT ( 'NONE',  ( -75.87500000409677625, 55.00000000000000000, -24.99999999999999645 ) ) ;
#10284=CARTESIAN_POINT ( 'NONE',  ( -77.00000000000000000, 55.00000000000000000, -24.99999999999999645 ) ) ;
#10285=VECTOR ( 'NONE', #4442, 1000.000000000000000 ) ;
#10288=ORIENTED_EDGE ( 'NONE', *, *, #9081, .F. ) ;
#10293=CARTESIAN_POINT ( 'NONE',  ( -23.67934118466866877, 78.62819164648935555, 8.208188635330966321 ) ) ;
#10296=CARTESIAN_POINT ( 'NONE',  ( -77.56250000409679046, 37.32233047033631124, -17.67766952966368166 ) ) ;
#10298=( LENGTH_UNIT ( ) NAMED_UNIT ( * ) SI_UNIT ( .MILLI., .METRE. ) );
#10301=CARTESIAN_POINT ( 'NONE',  ( -71.53052369147287948, 77.35376373433385311, 12.90594309674112772 ) ) ;
#10304=ORIENTED_EDGE ( 'NONE', *, *, #9294, .T. ) ;
#10305=CARTESIAN_POINT ( 'NONE',  ( -74.46875000000008527, 30.00000000000014921, 10.35533905932733489 ) ) ;
#10311=CARTESIAN_POINT ( 'NONE',  ( -72.96875000000007105, 30.00000000000015277, 10.35533905932733312 ) ) ;
#10315=ORIENTED_EDGE ( 'NONE', *, *, #10174, .T. ) ;
#10320=CARTESIAN_POINT ( 'NONE',  ( -75.12500000204838102, 29.18810118750000626, -10.69163855873949309 ) ) ;
#10321=EDGE_CURVE ( 'NONE', #546, #8432, #10957, .T. ) ;
#10324=CYLINDRICAL_SURFACE ( 'NONE', #10359, 24.99999999999999645 ) ;
#10328=CARTESIAN_POINT ( 'NONE',  ( -72.03125000204839523, 36.74823131438024859, -18.25176868561973720 ) ) ;
#10329=CARTESIAN_POINT ( 'NONE',  ( -72.59375000409677625, 80.00000000000001421, -10.35533905932737753 ) ) ;
#10336=EDGE_CURVE ( 'NONE', #193, #6797, #2496, .T. ) ;
#10337=VECTOR ( 'NONE', #9662, 1000.000000000000000 ) ;
#10339=CARTESIAN_POINT ( 'NONE',  ( 36.99999999999999289, 55.00000000000000000, 5.249999999999998224 ) ) ;
#10340=ORIENTED_EDGE ( 'NONE', *, *, #1143, .F. ) ;
#10344=CARTESIAN_POINT ( 'NONE',  ( -77.09375000000004263, 44.64466094067264379, -24.99999999999989697 ) ) ;
#10347=CARTESIAN_POINT ( 'NONE',  ( -76.25000000000000000, 55.00000000000000000, 24.99999999999999645 ) ) ;
#10353=CARTESIAN_POINT ( 'NONE',  ( 36.99999999999999289, 55.00000000000000000, 0.000000000000000000 ) ) ;
#10354=CARTESIAN_POINT ( 'NONE',  ( -14.94198242393282605, 71.73612833094152563, 18.58153189695169161 ) ) ;
#10357=CARTESIAN_POINT ( 'NONE',  ( -71.34302368722833876, 77.35376350879521112, 12.90594348738575903 ) ) ;
#10359=AXIS2_PLACEMENT_3D ( 'NONE', #3983, #2907, #7527 ) ;
#10361=CARTESIAN_POINT ( 'NONE',  ( 20.68439517297596453, 76.14615934997016211, -13.34036362221765692 ) ) ;
#10364=( BOUNDED_CURVE ( )  B_SPLINE_CURVE ( 2, ( #6461, #10214, #2975, #147, #5679, #7417, #9320, #9144, #1951 ),
 .UNSPECIFIED., .F., .T. ) 
 B_SPLINE_CURVE_WITH_KNOTS ( ( 3, 2, 2, 2, 3 ),
 ( 0.5833333333333338144, 0.6041666666666670737, 0.6250000000000004441, 0.6458333333333339255, 0.6666666666666671848 ),
 .UNSPECIFIED. ) 
 CURVE ( )  GEOMETRIC_REPRESENTATION_ITEM ( )  RATIONAL_B_SPLINE_CURVE ( ( 0.9999999999999983347, 0.9238795325112884038, 1.000000000000000000, 0.9238795325112867385, 1.000000000000000000, 0.9238795325112867385, 1.000000000000000000, 0.9238795325112847401, 1.000000000000001998 ) ) 
 REPRESENTATION_ITEM ( '' )  );
#10368=CARTESIAN_POINT ( 'NONE',  ( -72.68750000000000000, 37.32233047033631124, -17.67766952966368166 ) ) ;
#10370=PLANE ( 'NONE',  #1921 ) ;
#10378=CARTESIAN_POINT ( 'NONE',  ( -77.18750000204838102, 44.30836144126052289, 25.81189881250000795 ) ) ;
#10381=CARTESIAN_POINT ( 'NONE',  ( -74.28125000204839523, 73.25176868561975141, 18.25176868561974075 ) ) ;
#10393=CARTESIAN_POINT ( 'NONE',  ( -15.00000000000000000, -30.00000000000000000, -10.00000000000000000 ) ) ;
#10399=VECTOR ( 'NONE', #8682, 1000.000000000000000 ) ;
#10401=LINE ( 'NONE', #11296, #10542 ) ;
#10408=FACE_BOUND ( 'NONE', #6882, .T. ) ;
#10409=EDGE_CURVE ( 'NONE', #10526, #1709, #7449, .T. ) ;
#10410=CARTESIAN_POINT ( 'NONE',  ( -77.93750000204838102, 44.30836144126049447, -25.81189881249999019 ) ) ;
#10411=CARTESIAN_POINT ( 'NONE',  ( 39.99999999999999289, 55.00000000000000000, 0.000000000000000000 ) ) ;
#10414=CARTESIAN_POINT ( 'NONE',  ( -74.00000000204840944, 44.30836144126053000, 25.81189881250000795 ) ) ;
#10421=ORIENTED_EDGE ( 'NONE', *, *, #6831, .T. ) ;
#10422=CARTESIAN_POINT ( 'NONE',  ( -73.06250000000000000, 37.32233047033631124, 17.67766952966369232 ) ) ;
#10427=LINE ( 'NONE', #1267, #9594 ) ;
#10430=CARTESIAN_POINT ( 'NONE',  ( 7.004752486429524083, 66.69611028691875276, -18.63618820634359352 ) ) ;
#10431=CARTESIAN_POINT ( 'NONE',  ( -79.53125000204838102, 55.00000000000000000, -25.81189881249999729 ) ) ;
#10434=CARTESIAN_POINT ( 'NONE',  ( -74.93750000204839523, 44.30836144126050158, -25.81189881249999374 ) ) ;
#10444=ADVANCED_FACE ( 'NONE', ( #6489 ), #4926, .T. ) ;
#10447=LINE ( 'NONE', #10393, #6499 ) ;
#10448=CARTESIAN_POINT ( 'NONE',  ( 39.99999999999999289, 55.00000000000000000, 24.99999999999999645 ) ) ;
#10455=AXIS2_PLACEMENT_3D ( 'NONE', #633, #7396, #1537 ) ;
#10464=CARTESIAN_POINT ( 'NONE',  ( -78.87500000204839523, 80.81189881250000440, 10.69163855873948243 ) ) ;
#10465=CARTESIAN_POINT ( 'NONE',  ( -76.06250000000005684, 37.32233047033638940, 17.67766952966361771 ) ) ;
#10467=ORIENTED_EDGE ( 'NONE', *, *, #1168, .F. ) ;
#10468=CARTESIAN_POINT ( 'NONE',  ( -78.12500000409677625, 55.00000000000000000, 24.99999999999999645 ) ) ;
#10477=VECTOR ( 'NONE', #1856, 1000.000000000000000 ) ;
#10478=VERTEX_POINT ( 'NONE', #3963 ) ;
#10480=CARTESIAN_POINT ( 'NONE',  ( -72.40625000000000000, 65.35533905932737753, -24.99999999999999645 ) ) ;
#10486=DIRECTION ( 'NONE',  ( 0.000000000000000000, 1.000000000000000000, 0.000000000000000000 ) ) ;
#10489=CARTESIAN_POINT ( 'NONE',  ( 16.75908867079492737, 72.98228652723742016, 12.73316312262223171 ) ) ;
#10490=CARTESIAN_POINT ( 'NONE',  ( -77.46875000204839523, 73.25176868561975141, 18.25176868561974075 ) ) ;
#10495=CARTESIAN_POINT ( 'NONE',  ( -79.53125000000001421, 79.99999999999998579, 10.35533905932735799 ) ) ;
#10498=VECTOR ( 'NONE', #2369, 1000.000000000000000 ) ;
#10499=DIRECTION ( 'NONE',  ( 1.000000000000000000, 0.000000000000000000, 0.000000000000000000 ) ) ;
#10500=EDGE_LOOP ( 'NONE', ( #7944, #6234, #4901, #7535 ) ) ;
#10507=CARTESIAN_POINT ( 'NONE',  ( -15.00000000000000355, 5.000000000000000000, 30.00000000000000711 ) ) ;
#10520=DIRECTION ( 'NONE',  ( -1.000000000000000000, -0.000000000000000000, -0.000000000000000000 ) ) ;
#10522=CARTESIAN_POINT ( 'NONE',  ( -74.46875000204839523, 80.81189881250000440, -1.580522963032174394E-15 ) ) ;
#10523=CARTESIAN_POINT ( 'NONE',  ( -16.16012453410070293, 72.62154289115962058, 17.74408479697386554 ) ) ;
#10525=CIRCLE ( 'NONE', #6917, 30.57961884250791940 ) ;
#10526=VERTEX_POINT ( 'NONE', #178 ) ;
#10527=CARTESIAN_POINT ( 'NONE',  ( -72.78125000409679046, 65.35533905932737753, -24.99999999999999645 ) ) ;
#10528=DIRECTION ( 'NONE',  ( 0.000000000000000000, 0.000000000000000000, 1.000000000000000000 ) ) ;
#10529=VERTEX_POINT ( 'NONE', #8462 ) ;
#10535=CARTESIAN_POINT ( 'NONE',  ( 14.99999999999999645, 0.000000000000000000, 10.00000000000000178 ) ) ;
#10542=VECTOR ( 'NONE', #11114, 1000.000000000000000 ) ;
#10543=CARTESIAN_POINT ( 'NONE',  ( -75.03125000000000000, 80.00000000000001421, 10.35533905932737397 ) ) ;
#10544=CARTESIAN_POINT ( 'NONE',  ( -15.00000000000000000, -30.00000000000000000, -10.00000000000000000 ) ) ;
#10546=ORIENTED_EDGE ( 'NONE', *, *, #6989, .T. ) ;
#10554=CARTESIAN_POINT ( 'NONE',  ( 21.49621555244012328, 76.81665687444413493, 2.927878090024194968 ) ) ;
#10562=VERTEX_POINT ( 'NONE', #3720 ) ;
#10563=LINE ( 'NONE', #3263, #889 ) ;
#10580=CARTESIAN_POINT ( 'NONE',  ( -76.71875000204839523, 29.18810118750000271, 4.741568889096522788E-15 ) ) ;
#10585=CARTESIAN_POINT ( 'NONE',  ( -71.00000000409677625, 80.00000000000000000, -1.530808498934191324E-15 ) ) ;
#10587=CARTESIAN_POINT ( 'NONE',  ( -71.93750000409677625, 37.32233047033631124, 17.67766952966369232 ) ) ;
#10594=CARTESIAN_POINT ( 'NONE',  ( -73.15625000000000000, 44.64466094067262958, 25.00000000000001066 ) ) ;
#10596=ORIENTED_EDGE ( 'NONE', *, *, #10695, .T. ) ;
#10602=CARTESIAN_POINT ( 'NONE',  ( 9.487511670936607189, 67.96374653773119690, 17.79157655645022373 ) ) ;
#10614=EDGE_CURVE ( 'NONE', #2344, #3830, #7943, .T. ) ;
#10619=CARTESIAN_POINT ( 'NONE',  ( -77.18750000204838102, 44.30836144126053000, 25.81189881250000795 ) ) ;
#10623=DIRECTION ( 'NONE',  ( -1.000000000000000000, -0.000000000000000000, -0.000000000000000000 ) ) ;
#10630=VECTOR ( 'NONE', #3363, 1000.000000000000000 ) ;
#10631=CARTESIAN_POINT ( 'NONE',  ( 0.000000000000000000, 5.000000000000000000, 0.000000000000000000 ) ) ;
#10633=ADVANCED_FACE ( 'NONE', ( #11317 ), #5888, .T. ) ;
#10637=CARTESIAN_POINT ( 'NONE',  ( 14.99999999999999645, 0.000000000000000000, 30.00000000000000711 ) ) ;
#10638=DIRECTION ( 'NONE',  ( -1.000000000000000000, -0.000000000000000000, -0.000000000000000000 ) ) ;
#10639=CARTESIAN_POINT ( 'NONE',  ( -71.37500000409677625, 55.00000000000000000, -24.99999999999999645 ) ) ;
#10642=VERTEX_POINT ( 'NONE', #2220 ) ;
#10650=AXIS2_PLACEMENT_3D ( 'NONE', #9571, #2144, #1368 ) ;
#10651=CARTESIAN_POINT ( 'NONE',  ( -77.09375000204839523, 36.74823131438026280, 18.25176868561974786 ) ) ;
#10653=AXIS2_PLACEMENT_3D ( 'NONE', #4349, #2242, #3323 ) ;
#10657=ORIENTED_EDGE ( 'NONE', *, *, #8583, .F. ) ;
#10665=CARTESIAN_POINT ( 'NONE',  ( -74.75000000204838102, 80.81189881250000440, -10.69163855873948954 ) ) ;
#10676=DIRECTION ( 'NONE',  ( -1.000000000000000000, -0.000000000000000000, 0.000000000000000000 ) ) ;
#10680=CARTESIAN_POINT ( 'NONE',  ( -77.00000000204838102, 29.18810118750000981, 10.69163855873950020 ) ) ;
#10684=VECTOR ( 'NONE', #3669, 1000.000000000000000 ) ;
#10694=ORIENTED_EDGE ( 'NONE', *, *, #3520, .T. ) ;
#10695=EDGE_CURVE ( 'NONE', #5411, #5255, #8765, .T. ) ;
#10702=CARTESIAN_POINT ( 'NONE',  ( -71.84375000409677625, 30.00000000000001421, 10.35533905932739174 ) ) ;
#10710=AXIS2_PLACEMENT_3D ( 'NONE', #8175, #10676, #9845 ) ;
#10713=CARTESIAN_POINT ( 'NONE',  ( -76.62500000204839523, 44.30836144126050158, -25.81189881249999374 ) ) ;
#10724=AXIS2_PLACEMENT_3D ( 'NONE', #4385, #6017, #6973 ) ;
#10731=LINE ( 'NONE', #1630, #5186 ) ;
#10732=CARTESIAN_POINT ( 'NONE',  ( -71.99927362086853577, 76.65063509461015201, 12.50000000000143352 ) ) ;
#10736=ORIENTED_EDGE ( 'NONE', *, *, #10001, .T. ) ;
#10738=( BOUNDED_CURVE ( )  B_SPLINE_CURVE ( 2, ( #5463, #892, #3665, #7330, #2533, #10955, #6426, #8941, #1571 ),
 .UNSPECIFIED., .F., .T. ) 
 B_SPLINE_CURVE_WITH_KNOTS ( ( 3, 2, 2, 2, 3 ),
 ( 0.07919667986333785159, 0.09899957127346223351, 0.1188024626835866154, 0.1386053540937109974, 0.1584082455038353654 ),
 .UNSPECIFIED. ) 
 CURVE ( )  GEOMETRIC_REPRESENTATION_ITEM ( )  RATIONAL_B_SPLINE_CURVE ( ( 0.9999999999999998890, 0.9238795325112866275, 0.9999999999999998890, 0.9238795325112866275, 0.9999999999999998890, 0.9238795325112866275, 0.9999999999999998890, 0.9238795325113071666, 0.9999999999999793499 ) ) 
 REPRESENTATION_ITEM ( '' )  );
#10743=CARTESIAN_POINT ( 'NONE',  ( -76.15625000204838102, 80.81189881250000440, -1.580522963032174394E-15 ) ) ;
#10747=ORIENTED_EDGE ( 'NONE', *, *, #11621, .T. ) ;
#10754=DIRECTION ( 'NONE',  ( 0.000000000000000000, -1.000000000000000000, 0.000000000000000000 ) ) ;
#10757=EDGE_CURVE ( 'NONE', #5487, #4040, #10854, .T. ) ;
#10759=CARTESIAN_POINT ( 'NONE',  ( -74.09375000409676204, 80.00000000000001421, -10.35533905932737753 ) ) ;
#10761=CARTESIAN_POINT ( 'NONE',  ( -15.00000000000000000, 55.00000000000000000, 20.00000000000000000 ) ) ;
#10766=CARTESIAN_POINT ( 'NONE',  ( -78.78125000409680467, 65.35533905932737753, -24.99999999999999645 ) ) ;
#10771=CARTESIAN_POINT ( 'NONE',  ( -75.59375000204839523, 36.74823131438026280, 18.25176868561974786 ) ) ;
#10776=CARTESIAN_POINT ( 'NONE',  ( 13.04220382236630726, 70.42307724981912997, 19.68376297946718267 ) ) ;
#10778=AXIS2_PLACEMENT_3D ( 'NONE', #9457, #10520, #465 ) ;
#10783=ORIENTED_EDGE ( 'NONE', *, *, #5065, .T. ) ;
#10797=CARTESIAN_POINT ( 'NONE',  ( -77.65625000204838102, 80.81189881250000440, -1.580522963032174394E-15 ) ) ;
#10799=ORIENTED_EDGE ( 'NONE', *, *, #11404, .T. ) ;
#10803=( BOUNDED_SURFACE ( )  B_SPLINE_SURFACE ( 1, 2, ( 
 ( #8153, #1849, #1011, #7441, #6370, #2878, #9277, #949, #168, #4735, #1910, #1738, #4671, #10109, #2815, #8324, #4614, #10895, #105, #6483, #1069, #3600, #2760, #8270, #9996, #3773, #2642, #827, #44, #5458, #6421, #6308, #11067, #6545, #9942, #5517, #8390, #3839, #5403, #3712, #7376, #9106, #2704, #10835, #9051, #4500, #886, #11794, #4561, #8212, #7265, #11847, #3658, #10950, #10051, #11003, #6844, #10414, #8510, #9341, #9401, #292, #6785, #2028, #2090, #4919, #4860, #6727, #2214, #5764, #3955, #5703, #2997, #9583, #3897, #8632, #4980, #2154, #3056, #5880, #11184, #7617, #9523, #9463, #4797, #1196, #10357 ),
 ( #8571, #3174, #10234, #5825, #11245, #5942, #7560, #350, #10468, #1129, #1249, #1313, #4077, #412, #10296, #2268, #4016, #7674, #8453, #11309, #3119, #6666, #11365, #5041, #7734, #1379, #8688, #470, #6607, #7503, #233, #11127, #2941, #7910, #5270, #1549, #6960, #5153, #8807, #4371, #584, #1434, #8744, #8023, #2385, #2450, #3472, #9638, #527, #699, #11539, #10759, #6061, #8917, #4305, #9696, #6898, #11421, #5098, #11661, #4190, #5214, #7963, #6116, #4251, #10527, #4127, #7850, #7137, #2335, #6005, #1603, #11479, #3290, #1493, #10702, #2568, #2515, #8864, #6235, #644, #9865, #9750, #3343, #10585, #11599, #3404 ) ),
 .UNSPECIFIED., .F., .F., .T. ) 
 B_SPLINE_SURFACE_WITH_KNOTS ( ( 2, 2 ),
 ( 3, 2, 2, 2, 2, 2, 2, 2, 2, 2, 2, 2, 2, 2, 2, 2, 2, 2, 2, 2, 2, 2, 2, 2, 2, 2, 2, 2, 2, 2, 2, 2, 2, 2, 2, 2, 2, 2, 2, 2, 2, 2, 2, 3 ),
 ( 0.000000000000000000, 1.000000000000000000 ),
 ( 0.000000000000000000, 0.02083333333333333218, 0.04166666666666666435, 0.06250000000000000000, 0.08333333333333332871, 0.1041666666666666713, 0.1250000000000000000, 0.1458333333333333426, 0.1666666666666666574, 0.1875000000000000000, 0.2083333333333333426, 0.2291666666666666574, 0.2500000000000000000, 0.2708333333333333148, 0.2916666666666666852, 0.3125000000000000000, 0.3333333333333333148, 0.3541666666666666852, 0.3750000000000000000, 0.3958333333333333148, 0.4166666666666666852, 0.4375000000000000000, 0.4583333333333333148, 0.4791666666666666852, 0.5000000000000000000, 0.5208333333333333703, 0.5416666666666666297, 0.5625000000000000000, 0.5833333333333333703, 0.6041666666666666297, 0.6250000000000000000, 0.6458333333333333703, 0.6666666666666666297, 0.6875000000000000000, 0.7083333333333333703, 0.7291666666666666297, 0.7500000000000000000, 0.7708333333333333703, 0.7916666666666666297, 0.8125000000000000000, 0.8333333333333333703, 0.8541666666666666297, 0.8750000000000000000, 0.8888490476107191451 ),
 .UNSPECIFIED. ) 
 GEOMETRIC_REPRESENTATION_ITEM ( )  RATIONAL_B_SPLINE_SURFACE ( (
 ( 1.000000000000000000, 0.9238795325112867385, 1.000000000000000000, 0.9238795325112867385, 1.000000000000000000, 0.9238795325112867385, 1.000000000000000000, 0.9238795325112867385, 1.000000000000000000, 0.9238795325112867385, 1.000000000000000000, 0.9238795325112867385, 1.000000000000000000, 0.9238795325112867385, 1.000000000000000000, 0.9238795325112867385, 1.000000000000000000, 0.9238795325112867385, 1.000000000000000000, 0.9238795325112867385, 1.000000000000000000, 0.9238795325112867385, 1.000000000000000000, 0.9238795325112867385, 1.000000000000000000, 0.9238795325112867385, 1.000000000000000000, 0.9238795325112867385, 1.000000000000000000, 0.9238795325112867385, 1.000000000000000000, 0.9238795325112867385, 1.000000000000000000, 0.9238795325112867385, 1.000000000000000000, 0.9238795325112867385, 1.000000000000000000, 0.9238795325112867385, 1.000000000000000000, 0.9238795325112867385, 1.000000000000000000, 0.9238795325112867385, 1.000000000000000000, 0.9238795325112867385, 1.000000000000000000, 0.9238795325112867385, 1.000000000000000000, 0.9238795325112867385, 1.000000000000000000, 0.9238795325112867385, 1.000000000000000000, 0.9238795325112867385, 1.000000000000000000, 0.9238795325112867385, 1.000000000000000000, 0.9238795325112867385, 1.000000000000000000, 0.9238795325112867385, 1.000000000000000000, 0.9238795325112867385, 1.000000000000000000, 0.9238795325112867385, 1.000000000000000000, 0.9238795325112867385, 1.000000000000000000, 0.9238795325112867385, 1.000000000000000000, 0.9238795325112867385, 1.000000000000000000, 0.9238795325112867385, 1.000000000000000000, 0.9238795325112867385, 1.000000000000000000, 0.9238795325112867385, 1.000000000000000000, 0.9238795325112867385, 1.000000000000000000, 0.9238795325112867385, 1.000000000000000000, 0.9238795325112867385, 1.000000000000000000, 0.9238795325112867385, 1.000000000000000000, 0.9238795325112867385, 1.000000000000000000, 0.9493985930367334625, 0.9660721903170175207),
 ( 1.000000000000000000, 0.9238795325112867385, 1.000000000000000000, 0.9238795325112867385, 1.000000000000000000, 0.9238795325112867385, 1.000000000000000000, 0.9238795325112867385, 1.000000000000000000, 0.9238795325112867385, 1.000000000000000000, 0.9238795325112867385, 1.000000000000000000, 0.9238795325112867385, 1.000000000000000000, 0.9238795325112867385, 1.000000000000000000, 0.9238795325112867385, 1.000000000000000000, 0.9238795325112867385, 1.000000000000000000, 0.9238795325112867385, 1.000000000000000000, 0.9238795325112867385, 1.000000000000000000, 0.9238795325112867385, 1.000000000000000000, 0.9238795325112867385, 1.000000000000000000, 0.9238795325112867385, 1.000000000000000000, 0.9238795325112867385, 1.000000000000000000, 0.9238795325112867385, 1.000000000000000000, 0.9238795325112867385, 1.000000000000000000, 0.9238795325112867385, 1.000000000000000000, 0.9238795325112867385, 1.000000000000000000, 0.9238795325112867385, 1.000000000000000000, 0.9238795325112867385, 1.000000000000000000, 0.9238795325112867385, 1.000000000000000000, 0.9238795325112867385, 1.000000000000000000, 0.9238795325112867385, 1.000000000000000000, 0.9238795325112867385, 1.000000000000000000, 0.9238795325112867385, 1.000000000000000000, 0.9238795325112867385, 1.000000000000000000, 0.9238795325112867385, 1.000000000000000000, 0.9238795325112867385, 1.000000000000000000, 0.9238795325112867385, 1.000000000000000000, 0.9238795325112867385, 1.000000000000000000, 0.9238795325112867385, 1.000000000000000000, 0.9238795325112867385, 1.000000000000000000, 0.9238795325112867385, 1.000000000000000000, 0.9238795325112867385, 1.000000000000000000, 0.9238795325112867385, 1.000000000000000000, 0.9238795325112867385, 1.000000000000000000, 0.9238795325112867385, 1.000000000000000000, 0.9238795325112867385, 1.000000000000000000, 0.9238795325112867385, 1.000000000000000000, 0.9238795325112867385, 1.000000000000000000, 0.9493985930367334625, 0.9660721903170175207) ) ) 
 REPRESENTATION_ITEM ( '' )  SURFACE ( )  );
#10815=EDGE_CURVE ( 'NONE', #8716, #11173, #6363, .T. ) ;
#10819=DIRECTION ( 'NONE',  ( 0.000000000000000000, -0.000000000000000000, -1.000000000000000000 ) ) ;
#10831=CARTESIAN_POINT ( 'NONE',  ( -74.65625000204838102, 80.81189881250000440, -1.580522963032174394E-15 ) ) ;
#10835=CARTESIAN_POINT ( 'NONE',  ( -75.31250000204839523, 29.18810118750000981, 10.69163855873950020 ) ) ;
#10842=CARTESIAN_POINT ( 'NONE',  ( 2.400054171417768487E-15, 64.99605696851786263, -19.59792961213366169 ) ) ;
#10844=CARTESIAN_POINT ( 'NONE',  ( -74.09375000204839523, 36.74823131438026280, 18.25176868561974786 ) ) ;
#10854=CIRCLE ( 'NONE', #530, 22.00000000000000000 ) ;
#10855=CARTESIAN_POINT ( 'NONE',  ( -15.83487696431883762, 72.27984571272472181, -13.62867557726837475 ) ) ;
#10858=VERTEX_POINT ( 'NONE', #9990 ) ;
#10860=CARTESIAN_POINT ( 'NONE',  ( -75.78125000204838102, 55.00000000000000000, 25.81189881249999729 ) ) ;
#10874=VERTEX_POINT ( 'NONE', #7259 ) ;
#10882=CARTESIAN_POINT ( 'NONE',  ( -74.75000000000000000, 55.00000000000000000, 24.99999999999999645 ) ) ;
#10891=CARTESIAN_POINT ( 'NONE',  ( -74.46875000204839523, 73.25176868561975141, 18.25176868561974075 ) ) ;
#10894=ORIENTED_EDGE ( 'NONE', *, *, #9085, .F. ) ;
#10895=CARTESIAN_POINT ( 'NONE',  ( -77.75000000204839523, 65.69163855873948421, -25.81189881250000440 ) ) ;
#10896=VERTEX_POINT ( 'NONE', #708 ) ;
#10897=CARTESIAN_POINT ( 'NONE',  ( 22.02083420892270382, 77.24169289693605833, 11.42124585519064972 ) ) ;
#10900=CARTESIAN_POINT ( 'NONE',  ( -76.71875000409676204, 65.35533905932729226, 25.00000000000008527 ) ) ;
#10903=CARTESIAN_POINT ( 'NONE',  ( -78.12500000000004263, 79.99999999999992895, -1.530808498934187183E-15 ) ) ;
#10912=CARTESIAN_POINT ( 'NONE',  ( -3.611159399822559735, 65.46779913315577915, -19.35030201487227330 ) ) ;
#10913=AXIS2_PLACEMENT_3D ( 'NONE', #7381, #49, #8105 ) ;
#10918=VERTEX_POINT ( 'NONE', #3593 ) ;
#10920=CARTESIAN_POINT ( 'NONE',  ( -73.71875000204839523, 36.74823131438024859, -18.25176868561973720 ) ) ;
#10922=AXIS2_PLACEMENT_3D ( 'NONE', #1560, #4318, #1501 ) ;
#10923=ORIENTED_EDGE ( 'NONE', *, *, #2723, .F. ) ;
#10938=CARTESIAN_POINT ( 'NONE',  ( -76.71875000000004263, 79.99999999999990052, -10.35533905932733667 ) ) ;
#10947=CARTESIAN_POINT ( 'NONE',  ( -4.242132748603181014, 66.03411770982167184, -22.43350638257962615 ) ) ;
#10950=CARTESIAN_POINT ( 'NONE',  ( -74.37500000204838102, 80.81189881250001861, 10.69163855873948599 ) ) ;
#10955=CARTESIAN_POINT ( 'NONE',  ( -78.78125000000002842, 30.00000000000003553, -10.35533905932737042 ) ) ;
#10957=LINE ( 'NONE', #7272, #10477 ) ;
#10961=DIRECTION ( 'NONE',  ( 0.000000000000000000, 0.000000000000000000, 1.000000000000000000 ) ) ;
#10965=DIRECTION ( 'NONE',  ( -0.000000000000000000, -0.000000000000000000, -1.000000000000000000 ) ) ;
#10971=CARTESIAN_POINT ( 'NONE',  ( -78.40625000204839523, 36.74823131438026280, 18.25176868561974786 ) ) ;
#10980=ORIENTED_EDGE ( 'NONE', *, *, #9896, .T. ) ;
#10993=CARTESIAN_POINT ( 'NONE',  ( -75.12500000409677625, 55.00000000000000000, 24.99999999999999645 ) ) ;
#10998=DIRECTION ( 'NONE',  ( 1.000000000000000000, 0.000000000000000000, 0.000000000000000000 ) ) ;
#10999=CARTESIAN_POINT ( 'NONE',  ( -6.643805856392553721, 66.86877144058414046, -22.00652157144978105 ) ) ;
#11003=CARTESIAN_POINT ( 'NONE',  ( -74.18750000204839523, 65.69163855873949842, 25.81189881250000440 ) ) ;
#11005=CARTESIAN_POINT ( 'NONE',  ( 8.158495005360048680, 67.55745455422055556, 21.62097722686486279 ) ) ;
#11007=( GEOMETRIC_REPRESENTATION_CONTEXT ( 3 ) GLOBAL_UNCERTAINTY_ASSIGNED_CONTEXT ( ( #1062 ) ) GLOBAL_UNIT_ASSIGNED_CONTEXT ( ( #8594, #5116, #3190 ) ) REPRESENTATION_CONTEXT ( 'NONE', 'WORKASPACE' ) );
#11009=DIRECTION ( 'NONE',  ( 0.000000000000000000, 1.000000000000000000, 0.000000000000000000 ) ) ;
#11018=CARTESIAN_POINT ( 'NONE',  ( -6.986265722248286458, 66.68765601544015453, -18.64146191746018744 ) ) ;
#11029=CARTESIAN_POINT ( 'NONE',  ( -77.28125000204839523, 73.25176868561975141, 18.25176868561974075 ) ) ;
#11036=CARTESIAN_POINT ( 'NONE',  ( -72.12500000409677625, 55.00000000000000000, 24.99999999999999645 ) ) ;
#11048=DIRECTION ( 'NONE',  ( 0.000000000000000000, 0.000000000000000000, -1.000000000000000000 ) ) ;
#11057=CARTESIAN_POINT ( 'NONE',  ( -74.37500000409677625, 55.00000000000000000, -24.99999999999999645 ) ) ;
#11061=CARTESIAN_POINT ( 'NONE',  ( -72.21875000204838102, 36.74823131438024859, -18.25176868561973720 ) ) ;
#11062=FACE_OUTER_BOUND ( 'NONE', #5177, .T. ) ;
#11064=CARTESIAN_POINT ( 'NONE',  ( -1.724194960439331403, 65.52574505033150842, -22.67620946298737294 ) ) ;
#11067=CARTESIAN_POINT ( 'NONE',  ( -76.34375000204839523, 55.00000000000000000, -25.81189881249999729 ) ) ;
#11069=ORIENTED_EDGE ( 'NONE', *, *, #8953, .T. ) ;
#11070=PLANE ( 'NONE',  #7051 ) ;
#11077=AXIS2_PLACEMENT_3D ( 'NONE', #6404, #11830, #5499 ) ;
#11079=CARTESIAN_POINT ( 'NONE',  ( -74.37500000000008527, 30.00000000000013500, 4.592425496802549123E-15 ) ) ;
#11082=CARTESIAN_POINT ( 'NONE',  ( 39.99999999999999289, 55.00000000000000000, 24.99999999999999645 ) ) ;
#11084=CARTESIAN_POINT ( 'NONE',  ( -21.35532735205402943, 76.69866270122111018, -3.646780783107293811 ) ) ;
#11087=LINE ( 'NONE', #3078, #894 ) ;
#11092=CARTESIAN_POINT ( 'NONE',  ( -76.62500000204839523, 29.18810118750000626, -10.69163855873949309 ) ) ;
#11098=CARTESIAN_POINT ( 'NONE',  ( -73.43750000204839523, 44.30836144126049447, -25.81189881249999019 ) ) ;
#11099=CARTESIAN_POINT ( 'NONE',  ( -80.00000000000000000, 55.00000000000000000, 0.000000000000000000 ) ) ;
#11101=ORIENTED_EDGE ( 'NONE', *, *, #8439, .T. ) ;
#11108=CARTESIAN_POINT ( 'NONE',  ( -71.99927362086853577, 76.65063509461016622, 12.50000000000143352 ) ) ;
#11109=ORIENTED_EDGE ( 'NONE', *, *, #5660, .F. ) ;
#11114=DIRECTION ( 'NONE',  ( 0.000000000000000000, 1.000000000000000000, 0.000000000000000000 ) ) ;
#11118=ORIENTED_EDGE ( 'NONE', *, *, #9371, .F. ) ;
#11124=CARTESIAN_POINT ( 'NONE',  ( -19.44873419826854999, 75.15323065158862903, -14.79757583295479684 ) ) ;
#11127=CARTESIAN_POINT ( 'NONE',  ( -75.96875000409677625, 44.64466094067260826, -24.99999999999998934 ) ) ;
#11129=DIRECTION ( 'NONE',  ( 0.000000000000000000, 0.000000000000000000, -1.000000000000000000 ) ) ;
#11133=CARTESIAN_POINT ( 'NONE',  ( 39.99999999999999289, 55.00000000000000000, -22.00000000000000000 ) ) ;
#11140=CARTESIAN_POINT ( 'NONE',  ( -3.619482055381507024, 65.46993227710001406, 19.34915035418615048 ) ) ;
#11142=ORIENTED_EDGE ( 'NONE', *, *, #5708, .F. ) ;
#11148=CARTESIAN_POINT ( 'NONE',  ( -76.34375000204839523, 55.00000000000000000, -25.81189881249999729 ) ) ;
#11153=CIRCLE ( 'NONE', #831, 24.99999999999999645 ) ;
#11157=ORIENTED_EDGE ( 'NONE', *, *, #8000, .F. ) ;
#11166=DIRECTION ( 'NONE',  ( -1.000000000000000000, -0.000000000000000000, -0.000000000000000000 ) ) ;
#11171=CARTESIAN_POINT ( 'NONE',  ( -75.03125000409677625, 44.64466094067250168, 24.99999999999987566 ) ) ;
#11173=VERTEX_POINT ( 'NONE', #8385 ) ;
#11175=DIRECTION ( 'NONE',  ( 0.000000000000000000, 1.000000000000000000, 0.000000000000000000 ) ) ;
#11179=CARTESIAN_POINT ( 'NONE',  ( -19.18862861118784124, 74.94684730933501271, -15.07442433330465548 ) ) ;
#11184=CARTESIAN_POINT ( 'NONE',  ( -71.84375000204838102, 55.00000000000000000, -25.81189881249999729 ) ) ;
#11186=CARTESIAN_POINT ( 'NONE',  ( 7.761716740762911293, 67.37671573469675934, -21.72224607068988789 ) ) ;
#11190=CARTESIAN_POINT ( 'NONE',  ( 39.99999999999999289, 55.00000000000000000, -24.99999999999999645 ) ) ;
#11197=CARTESIAN_POINT ( 'NONE',  ( -74.56250000000008527, 37.32233047033641071, 17.67766952966359639 ) ) ;
#11202=CARTESIAN_POINT ( 'NONE',  ( -2.544240217464419196, 65.22984941951537508, 19.47702325593730066 ) ) ;
#11208=CARTESIAN_POINT ( 'NONE',  ( 36.99999999999999289, 55.00000000000000000, -5.249999999999998224 ) ) ;
#11211=CARTESIAN_POINT ( 'NONE',  ( -74.46875000204839523, 80.81189881250000440, -1.580522963032174394E-15 ) ) ;
#11214=CARTESIAN_POINT ( 'NONE',  ( -79.90625000000001421, 65.35533905932736332, -24.99999999999996803 ) ) ;
#11215=VECTOR ( 'NONE', #2035, 1000.000000000000000 ) ;
#11216=AXIS2_PLACEMENT_3D ( 'NONE', #10353, #10998, #6722 ) ;
#11224=AXIS2_PLACEMENT_3D ( 'NONE', #5788, #4821, #313 ) ;
#11233=LINE ( 'NONE', #10223, #9965 ) ;
#11234=FACE_BOUND ( 'NONE', #3704, .T. ) ;
#11238=CARTESIAN_POINT ( 'NONE',  ( -71.34302368722835297, 77.35376350879521112, 12.90594348738575903 ) ) ;
#11242=CARTESIAN_POINT ( 'NONE',  ( -25.22862615038675926, 79.94748894109862647, 1.675193470868706180 ) ) ;
#11245=CARTESIAN_POINT ( 'NONE',  ( -78.50000000409677625, 80.00000000000000000, -1.530808498934191324E-15 ) ) ;
#11256=CARTESIAN_POINT ( 'NONE',  ( -75.59375000000000000, 44.64466094067260826, -24.99999999999998934 ) ) ;
#11261=( BOUNDED_CURVE ( )  B_SPLINE_CURVE ( 2, ( #2123, #5851, #1219, #4886, #4049, #8537, #3986, #7646, #6757 ),
 .UNSPECIFIED., .F., .T. ) 
 B_SPLINE_CURVE_WITH_KNOTS ( ( 3, 2, 2, 2, 3 ),
 ( 0.08333333333333339810, 0.1041666666666667546, 0.1250000000000001110, 0.1458333333333334814, 0.1666666666666667962 ),
 .UNSPECIFIED. ) 
 CURVE ( )  GEOMETRIC_REPRESENTATION_ITEM ( )  RATIONAL_B_SPLINE_CURVE ( ( 0.9999999999999997780, 0.9238795325112869605, 1.000000000000000000, 0.9238795325112867385, 1.000000000000000000, 0.9238795325112867385, 1.000000000000000000, 0.9238795325112861834, 1.000000000000000444 ) ) 
 REPRESENTATION_ITEM ( '' )  );
#11267=DIRECTION ( 'NONE',  ( -1.000000000000000000, 0.000000000000000000, -0.000000000000000000 ) ) ;
#11268=CARTESIAN_POINT ( 'NONE',  ( -77.93750000204838102, 65.69163855873948421, -25.81189881250000084 ) ) ;
#11271=CARTESIAN_POINT ( 'NONE',  ( -73.06250000204840944, 80.81189881250001861, -10.69163855873949132 ) ) ;
#11279=CARTESIAN_POINT ( 'NONE',  ( -72.12500000204839523, 29.18810118750000626, -10.69163855873949132 ) ) ;
#11291=LINE ( 'NONE', #8493, #179 ) ;
#11296=CARTESIAN_POINT ( 'NONE',  ( 14.99999999999999645, -30.00000000000000000, -10.00000000000000000 ) ) ;
#11303=DIRECTION ( 'NONE',  ( 0.000000000000000000, 0.000000000000000000, -1.000000000000000000 ) ) ;
#11305=CARTESIAN_POINT ( 'NONE',  ( -75.12500000204838102, 29.18810118750000626, -10.69163855873949132 ) ) ;
#11306=FACE_OUTER_BOUND ( 'NONE', #2371, .T. ) ;
#11309=CARTESIAN_POINT ( 'NONE',  ( -77.09375000409677625, 80.00000000000001421, -10.35533905932737753 ) ) ;
#11317=FACE_OUTER_BOUND ( 'NONE', #1677, .T. ) ;
#11318=ORIENTED_EDGE ( 'NONE', *, *, #2521, .F. ) ;
#11319=CARTESIAN_POINT ( 'NONE',  ( -76.43750000000000000, 72.67766952966368876, 17.67766952966368521 ) ) ;
#11328=CARTESIAN_POINT ( 'NONE',  ( -74.75000000000000000, 55.00000000000000000, 24.99999999999999645 ) ) ;
#11329=CARTESIAN_POINT ( 'NONE',  ( -76.62500000204838102, 44.30836144126049447, -25.81189881249999019 ) ) ;
#11333=CARTESIAN_POINT ( 'NONE',  ( -78.87500000409677625, 55.00000000000000000, -24.99999999999999645 ) ) ;
#11339=ADVANCED_FACE ( 'NONE', ( #164, #1125 ), #4856, .F. ) ;
#11345=DIRECTION ( 'NONE',  ( 1.000000000000000000, 0.000000000000000000, 0.000000000000000000 ) ) ;
#11346=CARTESIAN_POINT ( 'NONE',  ( -75.96875000409676204, 44.64466094067271484, -25.00000000000010303 ) ) ;
#11353=FACE_OUTER_BOUND ( 'NONE', #8589, .T. ) ;
#11361=CARTESIAN_POINT ( 'NONE',  ( -76.81250000204839523, 29.18810118750000981, 10.69163855873950020 ) ) ;
#11365=CARTESIAN_POINT ( 'NONE',  ( -76.81250000409679046, 72.67766952966368876, 17.67766952966368521 ) ) ;
#11374=CARTESIAN_POINT ( 'NONE',  ( -78.12500000000000000, 80.00000000000000000, -1.530808498934191324E-15 ) ) ;
#11380=CARTESIAN_POINT ( 'NONE',  ( -73.25000000000000000, 55.00000000000000000, 24.99999999999999645 ) ) ;
#11384=CARTESIAN_POINT ( 'NONE',  ( 18.41262152147913156, 74.28295599064558985, 10.66131699734120275 ) ) ;
#11387=CARTESIAN_POINT ( 'NONE',  ( -74.84375000204839523, 55.00000000000000000, -25.81189881249999729 ) ) ;
#11397=CARTESIAN_POINT ( 'NONE',  ( 39.99999999999999289, 55.00000000000000000, 22.00000000000000000 ) ) ;
#11401=ORIENTED_EDGE ( 'NONE', *, *, #4460, .F. ) ;
#11404=EDGE_CURVE ( 'NONE', #5117, #2595, #1802, .T. ) ;
#11406=EDGE_CURVE ( 'NONE', #546, #1153, #706, .T. ) ;
#11415=CARTESIAN_POINT ( 'NONE',  ( -75.50000000204840944, 44.30836144126052289, 25.81189881250000795 ) ) ;
#11416=CARTESIAN_POINT ( 'NONE',  ( -8.150614517903754574, 67.55343220693646344, 21.62334187180388767 ) ) ;
#11421=CARTESIAN_POINT ( 'NONE',  ( -73.53125000409676204, 44.64466094067262958, 25.00000000000001066 ) ) ;
#11432=ORIENTED_EDGE ( 'NONE', *, *, #878, .T. ) ;
#11434=CARTESIAN_POINT ( 'NONE',  ( -73.71875000000000000, 80.00000000000001421, -10.35533905932737753 ) ) ;
#11442=CARTESIAN_POINT ( 'NONE',  ( 5.010510290115603560, 65.89460049710385192, -19.11356980082808832 ) ) ;
#11443=CARTESIAN_POINT ( 'NONE',  ( -79.43750000204838102, 65.69163855873948421, -25.81189881250000084 ) ) ;
#11445=CARTESIAN_POINT ( 'NONE',  ( -74.56250000204839523, 80.81189881250001861, -10.69163855873949132 ) ) ;
#11449=AXIS2_PLACEMENT_3D ( 'NONE', #10411, #2209, #2265 ) ;
#11460=DIRECTION ( 'NONE',  ( -1.000000000000000000, -0.000000000000000000, -0.000000000000000000 ) ) ;
#11474=CARTESIAN_POINT ( 'NONE',  ( -74.18750000204839523, 65.69163855873949842, 25.81189881250000084 ) ) ;
#11475=CARTESIAN_POINT ( 'NONE',  ( -23.80750660682828013, 78.73676915960464839, -7.856738918655103987 ) ) ;
#11479=CARTESIAN_POINT ( 'NONE',  ( -72.12500000409677625, 55.00000000000000000, 24.99999999999999645 ) ) ;
#11492=CARTESIAN_POINT ( 'NONE',  ( -77.37500000000000000, 30.00000000000000355, 4.592425496802573578E-15 ) ) ;
#11498=VERTEX_POINT ( 'NONE', #3988 ) ;
#11505=CARTESIAN_POINT ( 'NONE',  ( 3.626376041244185000, 65.46044694857717161, 19.35555878592614931 ) ) ;
#11506=CARTESIAN_POINT ( 'NONE',  ( -78.31250000204838102, 29.18810118750000626, -10.69163855873949132 ) ) ;
#11508=( BOUNDED_CURVE ( )  B_SPLINE_CURVE ( 2, ( #10993, #11171, #2986, #8313, #6652, #11838, #3648, #7315, #11057 ),
 .UNSPECIFIED., .F., .T. ) 
 B_SPLINE_CURVE_WITH_KNOTS ( ( 3, 2, 2, 2, 3 ),
 ( 0.4166666666666670182, 0.4375000000000003331, 0.4583333333333337034, 0.4791666666666670737, 0.5000000000000004441 ),
 .UNSPECIFIED. ) 
 CURVE ( )  GEOMETRIC_REPRESENTATION_ITEM ( )  RATIONAL_B_SPLINE_CURVE ( ( 0.9999999999999987788, 0.9238795325112879597, 1.000000000000000000, 0.9238795325112867385, 1.000000000000000000, 0.9238795325112867385, 1.000000000000000000, 0.9238795325112850731, 1.000000000000001554 ) ) 
 REPRESENTATION_ITEM ( '' )  );
#11522=CARTESIAN_POINT ( 'NONE',  ( -78.50000000204840944, 29.18810118750000981, 10.69163855873950020 ) ) ;
#11523=VERTEX_POINT ( 'NONE', #8778 ) ;
#11527=CARTESIAN_POINT ( 'NONE',  ( 39.99999999999999289, 55.00000000000000000, 0.000000000000000000 ) ) ;
#11535=CARTESIAN_POINT ( 'NONE',  ( -75.68750000204839523, 65.69163855873949842, 25.81189881250000084 ) ) ;
#11536=CARTESIAN_POINT ( 'NONE',  ( -75.78125000000005684, 30.00000000000011013, -10.35533905932734022 ) ) ;
#11539=CARTESIAN_POINT ( 'NONE',  ( -74.18750000409677625, 72.67766952966368876, -17.67766952966368876 ) ) ;
#11547=EDGE_CURVE ( 'NONE', #2344, #4746, #10563, .T. ) ;
#11548=CARTESIAN_POINT ( 'NONE',  ( -80.00000000000000000, 55.00000000000000000, 0.000000000000000000 ) ) ;
#11551=CARTESIAN_POINT ( 'NONE',  ( -76.34375000204839523, 73.25176868561975141, -18.25176868561974430 ) ) ;
#11560=CARTESIAN_POINT ( 'NONE',  ( -15.00000000000000000, -30.00000000000000000, 10.00000000000000000 ) ) ;
#11563=CARTESIAN_POINT ( 'NONE',  ( 7.641399616170716946, 67.00208548034325418, 18.44179151512062020 ) ) ;
#11581=CARTESIAN_POINT ( 'NONE',  ( -77.56250000204838102, 80.81189881250001861, 10.69163855873948599 ) ) ;
#11587=VECTOR ( 'NONE', #10499, 1000.000000000000000 ) ;
#11599=CARTESIAN_POINT ( 'NONE',  ( -70.93935441986300816, 80.00000000000001421, 6.698726263377743351 ) ) ;
#11613=CARTESIAN_POINT ( 'NONE',  ( -78.31250000204838102, 29.18810118750000626, -10.69163855873949309 ) ) ;
#11618=ORIENTED_EDGE ( 'NONE', *, *, #485, .F. ) ;
#11621=EDGE_CURVE ( 'NONE', #1153, #546, #8180, .T. ) ;
#11624=CARTESIAN_POINT ( 'NONE',  ( 21.66013690459276830, 76.95426865197336497, 1.464350659237193542 ) ) ;
#11628=DIRECTION ( 'NONE',  ( -1.000000000000000000, -0.000000000000000000, -0.000000000000000000 ) ) ;
#11637=ORIENTED_EDGE ( 'NONE', *, *, #3960, .F. ) ;
#11641=VECTOR ( 'NONE', #8468, 1000.000000000000000 ) ;
#11647=( BOUNDED_SURFACE ( )  B_SPLINE_SURFACE ( 1, 2, ( 
 ( #1979, #5525, #7451, #9175, #3906, #10121, #962, #8278, #53, #5594, #3722, #1019, #4681, #7514, #2040, #5648, #5714, #1139, #116, #3783, #11374, #2282, #4929, #4027, #3967, #5833, #7626, #6910, #11492, #303, #5958, #421, #4990, #4083, #8643, #8756, #4202, #7743, #11319, #3127, #5051, #1259, #9595, #2163, #3183, #8520, #7801, #11256, #3068, #3302, #3241, #9473, #2346, #10543, #7861, #6071, #538, #8585, #360, #5109, #6015, #1390, #7684, #1444, #9706, #2223, #9649, #11434, #6794, #6970, #4869, #4138, #6856, #10594, #10422, #2398, #6738, #5891, #10368, #9534, #1326, #10480, #8698, #481, #2461, #6249, #7148, #824, #9876 ),
 ( #8932, #2583, #1614, #1502, #7976, #9938, #11673, #4319, #9762, #4496, #3483, #6366, #8149, #11613, #5163, #8817, #598, #1562, #11789, #7028, #8993, #4262, #1672, #3415, #7920, #5341, #10651, #4444, #6129, #7206, #7090, #10713, #768, #8098, #11551, #2526, #711, #11734, #5280, #3355, #6192, #1735, #10771, #9825, #5227, #3596, #3534, #8875, #7262, #4382, #654, #8035, #10831, #2638, #10891, #6305, #5399, #9048, #2701, #41, #9102, #1968, #3655, #1066, #7320, #3836, #944, #7372, #4732, #6479, #883, #8320, #4668, #1126, #9220, #2993, #6604, #4611, #1788, #9993, #8450, #3709, #230, #4557, #8207, #5638, #10172, #1008, #6542 ) ),
 .UNSPECIFIED., .F., .F., .F. ) 
 B_SPLINE_SURFACE_WITH_KNOTS ( ( 2, 2 ),
 ( 3, 2, 2, 2, 2, 2, 2, 2, 2, 2, 2, 2, 2, 2, 2, 2, 2, 2, 2, 2, 2, 2, 2, 2, 2, 2, 2, 2, 2, 2, 2, 2, 2, 2, 2, 2, 2, 2, 2, 2, 2, 2, 2, 2, 3 ),
 ( 0.000000000000000000, 1.000000000000000000 ),
 ( 0.000000000000000000, 0.02083333333333333218, 0.04166666666666666435, 0.06250000000000000000, 0.08333333333333332871, 0.1041666666666666713, 0.1250000000000000000, 0.1458333333333333426, 0.1666666666666666574, 0.1875000000000000000, 0.2083333333333333426, 0.2291666666666666574, 0.2500000000000000000, 0.2708333333333333148, 0.2916666666666666852, 0.3125000000000000000, 0.3333333333333333148, 0.3541666666666666852, 0.3750000000000000000, 0.3958333333333333148, 0.4166666666666666852, 0.4375000000000000000, 0.4583333333333333148, 0.4791666666666666852, 0.5000000000000000000, 0.5208333333333333703, 0.5416666666666666297, 0.5625000000000000000, 0.5833333333333333703, 0.6041666666666666297, 0.6250000000000000000, 0.6458333333333333703, 0.6666666666666666297, 0.6875000000000000000, 0.7083333333333333703, 0.7291666666666666297, 0.7500000000000000000, 0.7708333333333333703, 0.7916666666666666297, 0.8125000000000000000, 0.8333333333333333703, 0.8541666666666666297, 0.8750000000000000000, 0.8888490471511721891, 0.8977375376226839343 ),
 .UNSPECIFIED. ) 
 GEOMETRIC_REPRESENTATION_ITEM ( )  RATIONAL_B_SPLINE_SURFACE ( (
 ( 1.000000000000000000, 0.9238795325112867385, 1.000000000000000000, 0.9238795325112867385, 1.000000000000000000, 0.9238795325112867385, 1.000000000000000000, 0.9238795325112867385, 1.000000000000000000, 0.9238795325112867385, 1.000000000000000000, 0.9238795325112867385, 1.000000000000000000, 0.9238795325112867385, 1.000000000000000000, 0.9238795325112867385, 1.000000000000000000, 0.9238795325112867385, 1.000000000000000000, 0.9238795325112867385, 1.000000000000000000, 0.9238795325112867385, 1.000000000000000000, 0.9238795325112867385, 1.000000000000000000, 0.9238795325112867385, 1.000000000000000000, 0.9238795325112867385, 1.000000000000000000, 0.9238795325112867385, 1.000000000000000000, 0.9238795325112867385, 1.000000000000000000, 0.9238795325112867385, 1.000000000000000000, 0.9238795325112867385, 1.000000000000000000, 0.9238795325112867385, 1.000000000000000000, 0.9238795325112867385, 1.000000000000000000, 0.9238795325112867385, 1.000000000000000000, 0.9238795325112867385, 1.000000000000000000, 0.9238795325112867385, 1.000000000000000000, 0.9238795325112867385, 1.000000000000000000, 0.9238795325112867385, 1.000000000000000000, 0.9238795325112867385, 1.000000000000000000, 0.9238795325112867385, 1.000000000000000000, 0.9238795325112867385, 1.000000000000000000, 0.9238795325112867385, 1.000000000000000000, 0.9238795325112867385, 1.000000000000000000, 0.9238795325112867385, 1.000000000000000000, 0.9238795325112867385, 1.000000000000000000, 0.9238795325112867385, 1.000000000000000000, 0.9238795325112867385, 1.000000000000000000, 0.9238795325112867385, 1.000000000000000000, 0.9238795325112867385, 1.000000000000000000, 0.9238795325112867385, 1.000000000000000000, 0.9238795325112867385, 1.000000000000000000, 0.9238795325112867385, 1.000000000000000000, 0.9238795325112867385, 1.000000000000000000, 0.9238795325112867385, 1.000000000000000000, 0.9238795325112867385, 1.000000000000000000, 0.9493985947158180005, 0.9660721892104719988, 0.9660721892104719988, 0.9660721892104719988),
 ( 1.000000000000000000, 0.9238795325112867385, 1.000000000000000000, 0.9238795325112867385, 1.000000000000000000, 0.9238795325112867385, 1.000000000000000000, 0.9238795325112867385, 1.000000000000000000, 0.9238795325112867385, 1.000000000000000000, 0.9238795325112867385, 1.000000000000000000, 0.9238795325112867385, 1.000000000000000000, 0.9238795325112867385, 1.000000000000000000, 0.9238795325112867385, 1.000000000000000000, 0.9238795325112867385, 1.000000000000000000, 0.9238795325112867385, 1.000000000000000000, 0.9238795325112867385, 1.000000000000000000, 0.9238795325112867385, 1.000000000000000000, 0.9238795325112867385, 1.000000000000000000, 0.9238795325112867385, 1.000000000000000000, 0.9238795325112867385, 1.000000000000000000, 0.9238795325112867385, 1.000000000000000000, 0.9238795325112867385, 1.000000000000000000, 0.9238795325112867385, 1.000000000000000000, 0.9238795325112867385, 1.000000000000000000, 0.9238795325112867385, 1.000000000000000000, 0.9238795325112867385, 1.000000000000000000, 0.9238795325112867385, 1.000000000000000000, 0.9238795325112867385, 1.000000000000000000, 0.9238795325112867385, 1.000000000000000000, 0.9238795325112867385, 1.000000000000000000, 0.9238795325112867385, 1.000000000000000000, 0.9238795325112867385, 1.000000000000000000, 0.9238795325112867385, 1.000000000000000000, 0.9238795325112867385, 1.000000000000000000, 0.9238795325112867385, 1.000000000000000000, 0.9238795325112867385, 1.000000000000000000, 0.9238795325112867385, 1.000000000000000000, 0.9238795325112867385, 1.000000000000000000, 0.9238795325112867385, 1.000000000000000000, 0.9238795325112867385, 1.000000000000000000, 0.9238795325112867385, 1.000000000000000000, 0.9238795325112867385, 1.000000000000000000, 0.9238795325112867385, 1.000000000000000000, 0.9238795325112867385, 1.000000000000000000, 0.9238795325112867385, 1.000000000000000000, 0.9238795325112867385, 1.000000000000000000, 0.9493985947158180005, 0.9660721892104719988, 0.9660721892104719988, 0.9660721892104719988) ) ) 
 REPRESENTATION_ITEM ( '' )  SURFACE ( )  );
#11658=DIRECTION ( 'NONE',  ( 0.000000000000000000, 0.000000000000000000, 1.000000000000000000 ) ) ;
#11661=CARTESIAN_POINT ( 'NONE',  ( -73.34375000409679046, 30.00000000000001421, 10.35533905932739174 ) ) ;
#11673=CARTESIAN_POINT ( 'NONE',  ( -78.96875000204839523, 73.25176868561975141, 18.25176868561974075 ) ) ;
#11681=AXIS2_PLACEMENT_3D ( 'NONE', #7553, #6537, #4009 ) ;
#11685=CIRCLE ( 'NONE', #4808, 22.00000000000000000 ) ;
#11687=CARTESIAN_POINT ( 'NONE',  ( -72.50000000204836681, 29.18810118750000981, 10.69163855873950020 ) ) ;
#11693=UNCERTAINTY_MEASURE_WITH_UNIT (LENGTH_MEASURE( 1.000000000000000082E-05 ), #10298, 'distance_accuracy_value', 'NONE');
#11701=ORIENTED_EDGE ( 'NONE', *, *, #3917, .T. ) ;
#11706=CARTESIAN_POINT ( 'NONE',  ( -78.12500000204838102, 44.30836144126050158, -25.81189881249999374 ) ) ;
#11727=ORIENTED_EDGE ( 'NONE', *, *, #11547, .T. ) ;
#11730=DIRECTION ( 'NONE',  ( 0.000000000000000000, -0.000000000000000000, 1.000000000000000000 ) ) ;
#11734=CARTESIAN_POINT ( 'NONE',  ( -76.06250000204839523, 80.81189881250001861, 10.69163855873948599 ) ) ;
#11739=CARTESIAN_POINT ( 'NONE',  ( 0.4285831363683495487, 65.42943686846955131, 22.72062601704910989 ) ) ;
#11742=CARTESIAN_POINT ( 'NONE',  ( -77.37500000409677625, 55.00000000000000000, -24.99999999999999645 ) ) ;
#11744=CARTESIAN_POINT ( 'NONE',  ( -74.18750000204838102, 44.30836144126052289, 25.81189881250000795 ) ) ;
#11750=DIRECTION ( 'NONE',  ( 1.000000000000000000, 0.000000000000000000, -0.000000000000000000 ) ) ;
#11757=CARTESIAN_POINT ( 'NONE',  ( -75.31250000204839523, 29.18810118750000626, -10.69163855873949309 ) ) ;
#11760=ORIENTED_EDGE ( 'NONE', *, *, #10614, .T. ) ;
#11763=EDGE_CURVE ( 'NONE', #4892, #847, #2777, .T. ) ;
#11767=ORIENTED_EDGE ( 'NONE', *, *, #4700, .T. ) ;
#11774=CARTESIAN_POINT ( 'NONE',  ( -70.87427368927673399, 76.65063840437989029, 12.49999426731031704 ) ) ;
#11789=CARTESIAN_POINT ( 'NONE',  ( -77.84375000204839523, 73.25176868561975141, -18.25176868561974430 ) ) ;
#11791=ORIENTED_EDGE ( 'NONE', *, *, #6586, .T. ) ;
#11794=CARTESIAN_POINT ( 'NONE',  ( -74.93750000204839523, 44.30836144126050158, -25.81189881249999374 ) ) ;
#11796=CARTESIAN_POINT ( 'NONE',  ( 16.17279400537643852, 72.62292825401752339, 17.77849829575843543 ) ) ;
#11803=( GEOMETRIC_REPRESENTATION_CONTEXT ( 3 ) GLOBAL_UNCERTAINTY_ASSIGNED_CONTEXT ( ( #4400 ) ) GLOBAL_UNIT_ASSIGNED_CONTEXT ( ( #4417, #5373, #7124 ) ) REPRESENTATION_CONTEXT ( 'NONE', 'WORKASPACE' ) );
#11811=CARTESIAN_POINT ( 'NONE',  ( -21.50191578866859388, 76.82143766378479199, 2.891252975302713857 ) ) ;
#11813=ORIENTED_EDGE ( 'NONE', *, *, #726, .F. ) ;
#11817=CARTESIAN_POINT ( 'NONE',  ( -77.46875000204839523, 80.81189881250000440, -1.580522963032174394E-15 ) ) ;
#11821=EDGE_CURVE ( 'NONE', #7813, #8716, #5719, .T. ) ;
#11823=CARTESIAN_POINT ( 'NONE',  ( -79.34375000204839523, 55.00000000000000000, -25.81189881249999729 ) ) ;
#11830=DIRECTION ( 'NONE',  ( -0.000000000000000000, -1.000000000000000000, -0.000000000000000000 ) ) ;
#11831=EDGE_LOOP ( 'NONE', ( #1963, #11637, #1531, #6735 ) ) ;
#11838=CARTESIAN_POINT ( 'NONE',  ( -74.65625000409679046, 30.00000000000000355, -10.35533905932738108 ) ) ;
#11847=CARTESIAN_POINT ( 'NONE',  ( -74.56250000204839523, 80.81189881250001861, -10.69163855873949132 ) ) ;
#11851=ADVANCED_FACE ( 'NONE', ( #3059 ), #11070, .F. ) ;
#11896=COLOUR_RGB('Off White',0.89,0.88,0.83);
#11897=FILL_AREA_STYLE_COLOUR('',#11896);
#11898=FILL_AREA_STYLE('',(#11897));
#11899=SURFACE_STYLE_FILL_AREA(#11898);
#11900=SURFACE_SIDE_STYLE('',(#11899));
#11901=SURFACE_STYLE_USAGE(.BOTH.,#11900);
#11902=PRESENTATION_STYLE_ASSIGNMENT((#11901));
ENDSEC;
END-ISO-10303-21;
